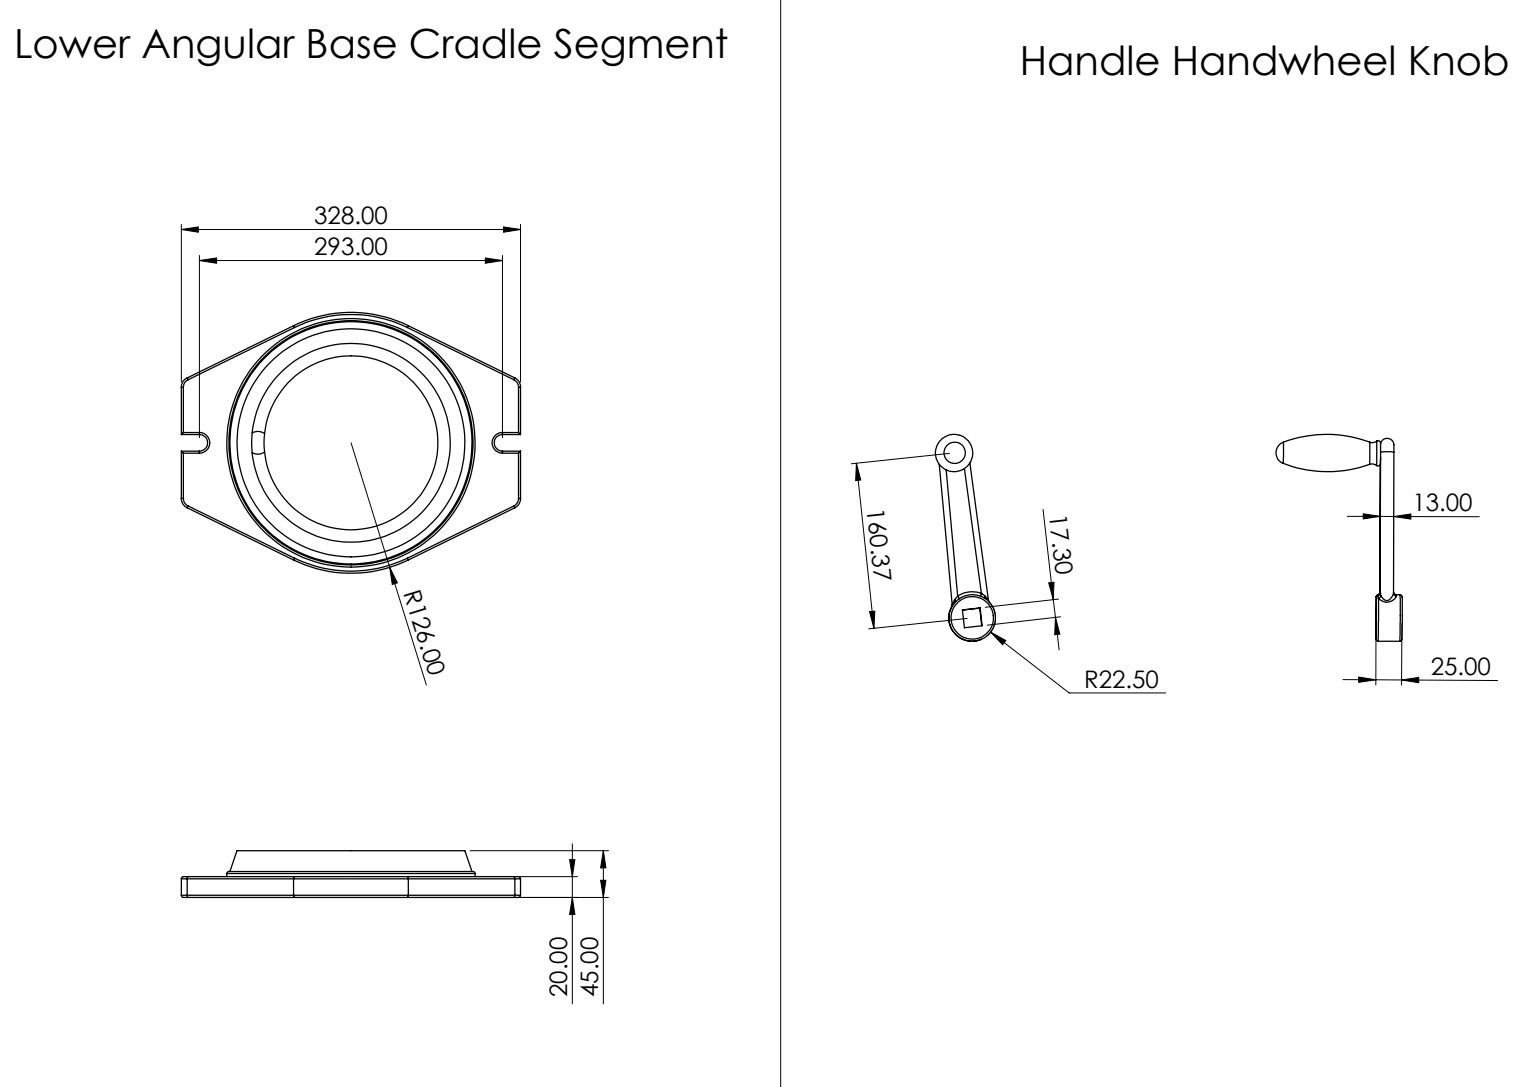
ISO-10303-21;
HEADER;
FILE_DESCRIPTION (('STEP AP214'),
    '1' );
FILE_NAME ('Handle Handwheel Knob.step',
    '2026-10-09T10:51:02',
    ( '' ),
    ( '' ),
    'SwSTEP 2.0',
    'SolidWorks 2026',
    '' );
FILE_SCHEMA (( 'AUTOMOTIVE_DESIGN' ));
ENDSEC;

DATA;
#6=CARTESIAN_POINT ( 'NONE',  ( -0.1662275214367944787, 327.2814318531398499, 311.3351636502816291 ) ) ;
#24=DIRECTION ( 'NONE',  ( 0.9935244165829104634, 0.1136188085379686713, 0.000000000000000000 ) ) ;
#26=CARTESIAN_POINT ( 'NONE',  ( -10.01057122740781402, 165.1012737418342056, 308.8014639846969089 ) ) ;
#27=EDGE_CURVE ( 'NONE', #4135, #17067, #5079, .T. ) ;
#41=CARTESIAN_POINT ( 'NONE',  ( 15.61516006123881795, 188.4668067408832144, 308.5202341143809690 ) ) ;
#52=CARTESIAN_POINT ( 'NONE',  ( 13.04681478898882219, 190.3009582326741622, 320.8498813576193243 ) ) ;
#55=CARTESIAN_POINT ( 'NONE',  ( 19.35063451732290929, 183.1639393726175058, 309.5798762404240847 ) ) ;
#63=CARTESIAN_POINT ( 'NONE',  ( -8.812762866403248907, 186.1645115285507188, 321.8620257335252859 ) ) ;
#87=CARTESIAN_POINT ( 'NONE',  ( -8.855655583235034101, 185.7709171679380802, 321.2465429934534313 ) ) ;
#92=DIRECTION ( 'NONE',  ( 0.9934404589540164476, 0.1135548637187057258, -0.01346653032743022095 ) ) ;
#97=CARTESIAN_POINT ( 'NONE',  ( -15.45047209318716419, 177.9595801977488634, 312.9923267615550344 ) ) ;
#100=B_SPLINE_CURVE_WITH_KNOTS ( 'NONE', 3,
 ( #8667, #13977, #4769, #10088, #15381, #20512, #13534 ),
 .UNSPECIFIED., .F., .F.,
 ( 4, 3, 4 ),
 ( -5.915969516749687466E-08, 0.000000000000000000, 2.978207829266907417E-05 ),
 .UNSPECIFIED. ) ;
#101=CARTESIAN_POINT ( 'NONE',  ( 17.83180013577688783, 184.4306634807684588, 307.6366520947308345 ) ) ;
#125=EDGE_CURVE ( 'NONE', #4735, #5612, #10337, .T. ) ;
#126=VERTEX_POINT ( 'NONE', #10448 ) ;
#128=CARTESIAN_POINT ( 'NONE',  ( 0.3194159855789066582, 327.3487718243365521, 314.2597695910868651 ) ) ;
#138=EDGE_CURVE ( 'NONE', #1183, #6442, #10411, .T. ) ;
#152=CARTESIAN_POINT ( 'NONE',  ( -28.12186643111994044, 324.0859723387359850, 311.7141148554663914 ) ) ;
#166=CARTESIAN_POINT ( 'NONE',  ( 14.63430001765469868, 189.2724070846429072, 308.1616490980433696 ) ) ;
#181=CARTESIAN_POINT ( 'NONE',  ( 15.18113699892158763, 188.8369998821271452, 308.3433818295962396 ) ) ;
#192=FACE_OUTER_BOUND ( 'NONE', #4432, .T. ) ;
#203=CARTESIAN_POINT ( 'NONE',  ( -8.718981069309306164, 185.8769606721263017, 321.2367416126799640 ) ) ;
#209=CARTESIAN_POINT ( 'NONE',  ( -16.46732747216173820, 164.3349221900030557, 301.8725943425079095 ) ) ;
#210=CARTESIAN_POINT ( 'NONE',  ( 15.90349308958513141, 168.0612899129591824, 307.9342904543644863 ) ) ;
#211=CARTESIAN_POINT ( 'NONE',  ( -13.46841022152523237, 180.7689078494431669, 321.2689861962914506 ) ) ;
#213=CARTESIAN_POINT ( 'NONE',  ( 20.69445389845595784, 181.8968845288082434, 314.6913679966366999 ) ) ;
#220=EDGE_CURVE ( 'NONE', #18203, #7136, #3541, .T. ) ;
#221=CARTESIAN_POINT ( 'NONE',  ( -17.10066205189340849, 316.2389990861104820, 322.8183011548654804 ) ) ;
#234=DIRECTION ( 'NONE',  ( -0.01292394549866745720, -0.005513023399720816918, -0.9999012842304692006 ) ) ;
#239=CARTESIAN_POINT ( 'NONE',  ( 21.90287145686899706, 168.7773271647431841, 315.3565719312696842 ) ) ;
#249=DIRECTION ( 'NONE',  ( 0.3101392564284310427, 0.9506461370142480494, -0.009250070373107139796 ) ) ;
#261=CARTESIAN_POINT ( 'NONE',  ( -28.28143568398816399, 324.0695986473149901, 312.1786345499324398 ) ) ;
#273=CARTESIAN_POINT ( 'NONE',  ( 19.91213793988244163, 183.5619383714575861, 314.9323046934921422 ) ) ;
#283=CARTESIAN_POINT ( 'NONE',  ( 19.70626577706693894, 182.8347090725441433, 310.2503944804881826 ) ) ;
#290=CARTESIAN_POINT ( 'NONE',  ( -9.470826101554981946, 187.1917151187963384, 321.2300099800097541 ) ) ;
#295=EDGE_LOOP ( 'NONE', ( #16677, #766, #19558, #3200 ) ) ;
#305=DIRECTION ( 'NONE',  ( 0.9506032891036977350, -0.3102281881984299550, -0.01057629388543066158 ) ) ;
#308=CARTESIAN_POINT ( 'NONE',  ( -22.02882225528089322, 319.7347194434814242, 320.5895957426023415 ) ) ;
#313=CARTESIAN_POINT ( 'NONE',  ( -10.06383400738342360, 187.4687485412983108, 321.1393786276795481 ) ) ;
#318=CARTESIAN_POINT ( 'NONE',  ( -13.33381189847107784, 183.5857969768588589, 309.7596506135559480 ) ) ;
#322=CARTESIAN_POINT ( 'NONE',  ( 18.31365161534814945, 168.3394720871181960, 308.5681747117120608 ) ) ;
#323=CARTESIAN_POINT ( 'NONE',  ( -14.60451153091767118, 179.2935387600311401, 317.4001766113444774 ) ) ;
#328=CARTESIAN_POINT ( 'NONE',  ( 11.85964614693714836, 187.7423844643599296, 304.8777488482054423 ) ) ;
#330=CARTESIAN_POINT ( 'NONE',  ( -9.841028579513169561, 187.8130746588807938, 321.1594247271215750 ) ) ;
#342=DIRECTION ( 'NONE',  ( 0.3101392564284315978, 0.9506461370142478273, -0.009250070373107145000 ) ) ;
#350=CARTESIAN_POINT ( 'NONE',  ( 0.2417370086904135351, 327.3338204178164688, 312.7560729848880214 ) ) ;
#360=CARTESIAN_POINT ( 'NONE',  ( -12.86548928906161571, 326.2291019854885121, 410.4442357137708086 ) ) ;
#372=CARTESIAN_POINT ( 'NONE',  ( -24.73308955485819283, 324.4589790655039110, 308.1131263010046837 ) ) ;
#382=ORIENTED_EDGE ( 'NONE', *, *, #15008, .F. ) ;
#385=CARTESIAN_POINT ( 'NONE',  ( 19.41596747074044060, 184.3392198334767329, 316.6735434663280557 ) ) ;
#399=CARTESIAN_POINT ( 'NONE',  ( 19.45541216839452048, 183.1297393420369417, 311.7642400163919660 ) ) ;
#408=CARTESIAN_POINT ( 'NONE',  ( -8.586490856789254167, 185.8024398487989686, 322.3033838124611634 ) ) ;
#431=CARTESIAN_POINT ( 'NONE',  ( -9.125680706444326162, 185.5535976647744860, 321.2577656795050984 ) ) ;
#435=CARTESIAN_POINT ( 'NONE',  ( -13.42037733046067238, 183.2664398413913887, 319.4772174752336582 ) ) ;
#439=CARTESIAN_POINT ( 'NONE',  ( -15.18250214363469119, 179.4876624324358261, 314.9100870799183554 ) ) ;
#504=CARTESIAN_POINT ( 'NONE',  ( 19.56830941617827335, 184.1114337889866874, 316.3329861247396479 ) ) ;
#518=CARTESIAN_POINT ( 'NONE',  ( 19.38763582148057907, 184.2660337520671590, 312.0117097956302814 ) ) ;
#538=CARTESIAN_POINT ( 'NONE',  ( 4.169604791867612015, 166.7785703876306513, 322.5944574396354483 ) ) ;
#553=CARTESIAN_POINT ( 'NONE',  ( -15.17867682233058524, 179.5161877312053207, 314.3080855853813205 ) ) ;
#556=DIRECTION ( 'NONE',  ( -0.9935244165829104634, -0.1136188085379686713, 0.000000000000000000 ) ) ;
#557=CARTESIAN_POINT ( 'NONE',  ( -15.13164630670634736, 179.6607342462910708, 313.7313605305386091 ) ) ;
#565=DIRECTION ( 'NONE',  ( 0.9934404589540163366, 0.1135548637187057675, -0.01346653032742958604 ) ) ;
#596=DIRECTION ( 'NONE',  ( -0.01292394549866742424, -0.005513023399720750999, -0.9999012842304693116 ) ) ;
#628=CARTESIAN_POINT ( 'NONE',  ( 18.96776859854577069, 184.9744126260587791, 317.4480445392455294 ) ) ;
#637=EDGE_CURVE ( 'NONE', #13714, #126, #15945, .T. ) ;
#642=CARTESIAN_POINT ( 'NONE',  ( -12.58664483627419095, 184.6272112293399630, 320.1917372557430213 ) ) ;
#658=CARTESIAN_POINT ( 'NONE',  ( -8.575531608407624518, 185.9784460181284089, 321.2405749393824976 ) ) ;
#662=CARTESIAN_POINT ( 'NONE',  ( -14.79896642201964418, 180.4272692235275315, 317.1363243735250421 ) ) ;
#664=CARTESIAN_POINT ( 'NONE',  ( -9.822685604078287724, 184.4798924047493642, 305.4113335104130442 ) ) ;
#667=ORIENTED_EDGE ( 'NONE', *, *, #3510, .T. ) ;
#674=CARTESIAN_POINT ( 'NONE',  ( 12.48881921303416398, 189.6164759944761897, 307.6758311242440982 ) ) ;
#730=CARTESIAN_POINT ( 'NONE',  ( 13.58462956591013615, 190.0212252665789094, 307.9296231100185537 ) ) ;
#734=MECHANICAL_DESIGN_GEOMETRIC_PRESENTATION_REPRESENTATION('',(#10620),#15073);
#746=CARTESIAN_POINT ( 'NONE',  ( 19.93997345945722799, 182.7315227521808936, 315.6546791933524787 ) ) ;
#766=ORIENTED_EDGE ( 'NONE', *, *, #125, .T. ) ;
#782=CARTESIAN_POINT ( 'NONE',  ( -9.048035673407987645, 185.0480505508585907, 307.9947944869788898 ) ) ;
#799=CARTESIAN_POINT ( 'NONE',  ( -14.20436985759224235, 179.8017517255571818, 320.1469751989672545 ) ) ;
#809=AXIS2_PLACEMENT_3D ( 'NONE', #3079, #12155, #12280 ) ;
#810=CARTESIAN_POINT ( 'NONE',  ( -8.564669286038160578, 185.5585649246744140, 306.1008109505842754 ) ) ;
#826=FACE_BOUND ( 'NONE', #21834, .T. ) ;
#838=CARTESIAN_POINT ( 'NONE',  ( -7.810477471022748475, 165.3506309087785553, 308.2453597648303685 ) ) ;
#846=CARTESIAN_POINT ( 'NONE',  ( 11.80591785795528104, 176.3657631373681056, 324.4430942173937638 ) ) ;
#854=B_SPLINE_CURVE_WITH_KNOTS ( 'NONE', 3,
 ( #18218, #21952, #12942, #4063, #16834, #5778, #2583 ),
 .UNSPECIFIED., .F., .F.,
 ( 4, 3, 4 ),
 ( 0.000000000000000000, 3.076089232684222182E-05, 3.082002332305258858E-05 ),
 .UNSPECIFIED. ) ;
#869=CARTESIAN_POINT ( 'NONE',  ( 18.86594229807002421, 185.1130985469481800, 317.5966198224662094 ) ) ;
#871=CARTESIAN_POINT ( 'NONE',  ( -3.415012492225389273, 157.2134297314921128, 324.7454257987990331 ) ) ;
#902=CARTESIAN_POINT ( 'NONE',  ( -12.78366430685853672, 181.7268150396907345, 309.3689789245013344 ) ) ;
#908=CARTESIAN_POINT ( 'NONE',  ( 11.85847056065619221, 187.7666840159210437, 305.2629551530478125 ) ) ;
#917=ORIENTED_EDGE ( 'NONE', *, *, #10755, .T. ) ;
#921=DIRECTION ( 'NONE',  ( 0.01292394549866727679, 0.005513023399720742325, 0.9999012842304692006 ) ) ;
#933=ORIENTED_EDGE ( 'NONE', *, *, #14009, .T. ) ;
#939=DIRECTION ( 'NONE',  ( -0.9934404589540161146, -0.1135548637187070442, 0.01346653032743022269 ) ) ;
#973=CARTESIAN_POINT ( 'NONE',  ( 24.23788345395560384, 168.9796455556705723, 299.3206640306223676 ) ) ;
#974=CARTESIAN_POINT ( 'NONE',  ( 17.82481991809018140, 186.4251367409188163, 318.7777147611763553 ) ) ;
#975=ADVANCED_FACE ( 'NONE', ( #17419 ), #6180, .T. ) ;
#981=DIRECTION ( 'NONE',  ( 0.1136178953597579561, -0.9935164314186356593, 0.004009283626633663132 ) ) ;
#1001=ADVANCED_FACE ( 'NONE', ( #19114 ), #14443, .F. ) ;
#1007=CARTESIAN_POINT ( 'NONE',  ( -11.47056600305460350, 183.0990483233374846, 308.4747080909204442 ) ) ;
#1010=CARTESIAN_POINT ( 'NONE',  ( 12.16442896649338223, 187.7168230983759543, 322.9757373289252200 ) ) ;
#1020=CARTESIAN_POINT ( 'NONE',  ( 12.21805463999710817, 187.9383611531376914, 322.3984907411651193 ) ) ;
#1067=CARTESIAN_POINT ( 'NONE',  ( -5.563703806604336499, 326.7005119474492290, 320.3383740725300299 ) ) ;
#1077=CARTESIAN_POINT ( 'NONE',  ( -17.21821209452539847, 315.6014859805258652, 330.9526324688387717 ) ) ;
#1083=CARTESIAN_POINT ( 'NONE',  ( 17.83341159513771856, 184.6399546625437722, 321.1738318148023836 ) ) ;
#1108=DIRECTION ( 'NONE',  ( -0.01292394549866727679, -0.005513023399720743192, -0.9999012842304693116 ) ) ;
#1109=CARTESIAN_POINT ( 'NONE',  ( 12.82628922073134170, 190.6145596806321407, 307.8497150165550238 ) ) ;
#1125=CARTESIAN_POINT ( 'NONE',  ( -13.62391555017718048, 183.0616513303022543, 310.0861352889502314 ) ) ;
#1140=DIRECTION ( 'NONE',  ( 0.3101392564284315978, 0.9506461370142478273, -0.009250070373107145000 ) ) ;
#1164=DIRECTION ( 'NONE',  ( -0.9934404589540163366, -0.1135548637187060866, 0.01346653032743036840 ) ) ;
#1183=VERTEX_POINT ( 'NONE', #1864 ) ;
#1205=ORIENTED_EDGE ( 'NONE', *, *, #10755, .F. ) ;
#1206=CARTESIAN_POINT ( 'NONE',  ( -16.17007672569239318, 164.4617217281966361, 324.8703238798086659 ) ) ;
#1208=CARTESIAN_POINT ( 'NONE',  ( 15.97866707245144902, 185.9292776491716381, 320.3317121505914997 ) ) ;
#1216=DIRECTION ( 'NONE',  ( -0.9934404589540162256, -0.1135548637187057258, 0.01346653032743021748 ) ) ;
#1224=ORIENTED_EDGE ( 'NONE', *, *, #8533, .T. ) ;
#1247=CARTESIAN_POINT ( 'NONE',  ( -9.772617557124883447, 188.0380679982199581, 308.1349344327151130 ) ) ;
#1248=EDGE_LOOP ( 'NONE', ( #10587, #8874 ) ) ;
#1255=CARTESIAN_POINT ( 'NONE',  ( 14.00406913739424830, 186.9630538133311006, 322.8218460857456193 ) ) ;
#1258=CARTESIAN_POINT ( 'NONE',  ( -0.3844496095692996329, 327.2789202713466352, 316.8969144942429921 ) ) ;
#1264=VERTEX_POINT ( 'NONE', #11052 ) ;
#1265=CARTESIAN_POINT ( 'NONE',  ( 12.29214828332425924, 188.1889653831995020, 322.0203645085242670 ) ) ;
#1281=ORIENTED_EDGE ( 'NONE', *, *, #11747, .T. ) ;
#1352=CARTESIAN_POINT ( 'NONE',  ( -10.17049351323417561, 187.7283718258219949, 308.1773159039984762 ) ) ;
#1357=CARTESIAN_POINT ( 'NONE',  ( 16.40873467035000033, 185.6567299720572635, 322.3321779654820602 ) ) ;
#1364=CARTESIAN_POINT ( 'NONE',  ( 13.70891000273312343, 189.9149113544312399, 320.7681615485908537 ) ) ;
#1368=FACE_OUTER_BOUND ( 'NONE', #21089, .T. ) ;
#1370=EDGE_CURVE ( 'NONE', #19478, #5262, #3205, .T. ) ;
#1374=CARTESIAN_POINT ( 'NONE',  ( -16.19592461668972661, 164.4506956813972067, 322.8705213113477726 ) ) ;
#1376=CARTESIAN_POINT ( 'NONE',  ( -12.01575389182678499, 182.4076787623492066, 322.7174846376903474 ) ) ;
#1378=CARTESIAN_POINT ( 'NONE',  ( -25.68841619517593955, 324.3516952872404318, 308.6004965912300690 ) ) ;
#1395=DIRECTION ( 'NONE',  ( 1.000000000000000000, 0.000000000000000000, 0.000000000000000000 ) ) ;
#1399=AXIS2_PLACEMENT_3D ( 'NONE', #7003, #12191, #342 ) ;
#1450=CARTESIAN_POINT ( 'NONE',  ( 13.01890817498768449, 190.3110758050131892, 320.8522954438618058 ) ) ;
#1472=CARTESIAN_POINT ( 'NONE',  ( 13.55544375494392817, 190.0065045115472913, 320.7925508485532760 ) ) ;
#1480=FACE_OUTER_BOUND ( 'NONE', #8854, .T. ) ;
#1503=ORIENTED_EDGE ( 'NONE', *, *, #12891, .T. ) ;
#1548=TOROIDAL_SURFACE ( 'NONE', #1905, 20.50000000000000355, 2.000000000000000000 ) ;
#1560=CARTESIAN_POINT ( 'NONE',  ( 11.78290328754079219, 187.7711080693391921, 304.8720351003711357 ) ) ;
#1578=SPHERICAL_SURFACE ( 'NONE', #14052, 11.00000000000000533 ) ;
#1594=CARTESIAN_POINT ( 'NONE',  ( 14.92693155316947262, 186.3292256045772604, 305.6379776027275170 ) ) ;
#1632=DIRECTION ( 'NONE',  ( -0.01292394549866727679, -0.005513023399720742325, -0.9999012842304692006 ) ) ;
#1634=ADVANCED_FACE ( 'NONE', ( #19289 ), #5393, .F. ) ;
#1648=DIRECTION ( 'NONE',  ( 0.1136178953597579561, -0.9935164314186356593, 0.004009283626633663132 ) ) ;
#1651=VECTOR ( 'NONE', #15859, 999.9999999999998863 ) ;
#1661=ORIENTED_EDGE ( 'NONE', *, *, #3227, .T. ) ;
#1675=( NAMED_UNIT ( * ) PLANE_ANGLE_UNIT ( ) SI_UNIT ( $, .RADIAN. ) );
#1678=CARTESIAN_POINT ( 'NONE',  ( 11.82873084905181749, 187.7848449878356405, 307.7666980689497791 ) ) ;
#1691=DIRECTION ( 'NONE',  ( -0.01292394549866745720, -0.005513023399720816918, -0.9999012842304692006 ) ) ;
#1708=CARTESIAN_POINT ( 'NONE',  ( 20.16650508637343719, 182.5115947525307263, 317.5179922051294739 ) ) ;
#1734=CARTESIAN_POINT ( 'NONE',  ( 0.3064506171779977084, 327.3432411309900090, 313.2566634950479170 ) ) ;
#1740=ORIENTED_EDGE ( 'NONE', *, *, #7164, .T. ) ;
#1754=CARTESIAN_POINT ( 'NONE',  ( -8.905365697803494740, 165.2773500475165065, 321.1137824091954940 ) ) ;
#1775=CARTESIAN_POINT ( 'NONE',  ( -14.02864438394168722, 325.7329298795136197, 320.4531201330285626 ) ) ;
#1780=CARTESIAN_POINT ( 'NONE',  ( 14.12971913360413367, 189.6478225779368358, 308.0282301501843563 ) ) ;
#1798=ORIENTED_EDGE ( 'NONE', *, *, #5168, .F. ) ;
#1802=CIRCLE ( 'NONE', #11336, 22.50000000000000000 ) ;
#1805=CARTESIAN_POINT ( 'NONE',  ( -12.19462927199251112, 185.2216277673267939, 320.4682053348163890 ) ) ;
#1811=DIRECTION ( 'NONE',  ( -0.7193492748294019190, 0.6946270388778962301, 0.005467875468530753770 ) ) ;
#1813=CARTESIAN_POINT ( 'NONE',  ( 15.81758052762976341, 168.0514417711093529, 307.9285322505227782 ) ) ;
#1814=CARTESIAN_POINT ( 'NONE',  ( -15.16114907798143285, 179.5344160342980615, 315.3037902903944314 ) ) ;
#1822=ADVANCED_FACE ( 'NONE', ( #192 ), #4319, .F. ) ;
#1840=CARTESIAN_POINT ( 'NONE',  ( 15.98577074487546312, 168.1231874004433280, 320.9410920942888197 ) ) ;
#1845=ORIENTED_EDGE ( 'NONE', *, *, #21487, .T. ) ;
#1864=CARTESIAN_POINT ( 'NONE',  ( -10.32533161609876871, 336.9590297039326288, 324.0204083566396207 ) ) ;
#1865=CARTESIAN_POINT ( 'NONE',  ( -7.642197790895533416, 165.4224147006813155, 321.2648411829814563 ) ) ;
#1882=CARTESIAN_POINT ( 'NONE',  ( 15.29545575833136084, 188.7412618571948144, 308.3876529512198204 ) ) ;
#1893=CARTESIAN_POINT ( 'NONE',  ( 13.03751462902003055, 190.3043364584464143, 320.8506857707324684 ) ) ;
#1896=CARTESIAN_POINT ( 'NONE',  ( 16.47746874666049166, 185.3946093038764218, 306.5053848239848548 ) ) ;
#1902=CARTESIAN_POINT ( 'NONE',  ( -9.012827358357725416, 186.4798162552521603, 321.5937060577796842 ) ) ;
#1905=AXIS2_PLACEMENT_3D ( 'NONE', #16224, #921, #17933 ) ;
#1911=AXIS2_PLACEMENT_3D ( 'NONE', #7697, #5853, #21910 ) ;
#1921=CARTESIAN_POINT ( 'NONE',  ( 12.33097383755215937, 187.6544282282688414, 322.9682109676994628 ) ) ;
#1927=CARTESIAN_POINT ( 'NONE',  ( -9.866459160504181369, 187.6519449355448046, 321.1574017861566972 ) ) ;
#1931=CARTESIAN_POINT ( 'NONE',  ( -15.16562817910661387, 179.5584899311543552, 314.0881026776677345 ) ) ;
#1934=CARTESIAN_POINT ( 'NONE',  ( -5.731715098087012628, 326.6288426432528240, 307.3396573775339107 ) ) ;
#1935=CARTESIAN_POINT ( 'NONE',  ( -13.94857819362903939, 180.2051281715647804, 318.6524844431677934 ) ) ;
#1937=CARTESIAN_POINT ( 'NONE',  ( 19.54762674317498039, 182.9836852283762880, 309.9251239444264456 ) ) ;
#1943=ORIENTED_EDGE ( 'NONE', *, *, #18930, .F. ) ;
#1965=CARTESIAN_POINT ( 'NONE',  ( 18.46443518240318937, 168.4037924862991815, 320.2340148651496179 ) ) ;
#1967=VERTEX_POINT ( 'NONE', #6596 ) ;
#1974=ORIENTED_EDGE ( 'NONE', *, *, #19587, .T. ) ;
#1988=CARTESIAN_POINT ( 'NONE',  ( -12.65694952506544801, 164.8377797042643635, 318.5015202093982225 ) ) ;
#1996=ORIENTED_EDGE ( 'NONE', *, *, #8299, .F. ) ;
#2008=AXIS2_PLACEMENT_3D ( 'NONE', #10847, #16145, #21169 ) ;
#2013=CARTESIAN_POINT ( 'NONE',  ( 18.63884989169994100, 183.8434042675073954, 310.4714192387435787 ) ) ;
#2031=CARTESIAN_POINT ( 'NONE',  ( 12.21332820092900739, 188.3547093575519682, 320.9587726345017131 ) ) ;
#2041=CARTESIAN_POINT ( 'NONE',  ( -14.34866974388063099, 181.6106202444769906, 311.1517963829039104 ) ) ;
#2044=CARTESIAN_POINT ( 'NONE',  ( -15.06566084134985850, 178.6016716131798887, 315.4181938385037256 ) ) ;
#2095=CARTESIAN_POINT ( 'NONE',  ( -26.01799913968005384, 324.3151495388358967, 308.8842677255468061 ) ) ;
#2115=CARTESIAN_POINT ( 'NONE',  ( 13.58411996604009886, 190.0215289310135347, 307.9295376775164073 ) ) ;
#2122=ORIENTED_EDGE ( 'NONE', *, *, #8358, .T. ) ;
#2133=CARTESIAN_POINT ( 'NONE',  ( 12.23821171205838709, 188.3449730651813638, 320.9566317594674274 ) ) ;
#2136=LINE ( 'NONE', #12384, #22139 ) ;
#2139=CARTESIAN_POINT ( 'NONE',  ( -9.651817171046198851, 185.0982321658034948, 321.2476234092152367 ) ) ;
#2144=CARTESIAN_POINT ( 'NONE',  ( -15.18631308743390740, 179.4818830208618010, 314.7524899164025101 ) ) ;
#2145=ORIENTED_EDGE ( 'NONE', *, *, #4888, .F. ) ;
#2148=CARTESIAN_POINT ( 'NONE',  ( -14.75085724879592419, 179.0757283420780936, 316.9950527168435883 ) ) ;
#2152=DIRECTION ( 'NONE',  ( -0.9934404589540165587, -0.1135548637187044907, 0.01346653032743213955 ) ) ;
#2186=TOROIDAL_SURFACE ( 'NONE', #5103, 17.29295143883736330, 7.000000000000003553 ) ;
#2188=AXIS2_PLACEMENT_3D ( 'NONE', #17082, #6393, #3045 ) ;
#2190=EDGE_CURVE ( 'NONE', #13179, #3953, #100, .T. ) ;
#2194=DIRECTION ( 'NONE',  ( -0.01292394549866745720, -0.005513023399720816918, -0.9999012842304692006 ) ) ;
#2197=CARTESIAN_POINT ( 'NONE',  ( -28.53175067654398234, 324.0509493238391201, 314.6508600760126910 ) ) ;
#2213=CARTESIAN_POINT ( 'NONE',  ( 17.50001040944635378, 186.7960900973744742, 319.0550816609377875 ) ) ;
#2219=DIRECTION ( 'NONE',  ( -0.9506868100732489557, 0.3101525256269085928, 0.000000000000000000 ) ) ;
#2225=CARTESIAN_POINT ( 'NONE',  ( 12.89457967643548031, 187.3266554051253081, 305.0022774674998800 ) ) ;
#2227=AXIS2_PLACEMENT_3D ( 'NONE', #13603, #8077, #20588 ) ;
#2232=DIRECTION ( 'NONE',  ( -0.01292394549866754394, -0.005513023399720772683, -0.9999012842304692006 ) ) ;
#2263=AXIS2_PLACEMENT_3D ( 'NONE', #17479, #234, #13903 ) ;
#2271=CARTESIAN_POINT ( 'NONE',  ( -15.06976562345401227, 178.6172216735134555, 313.9837765850090250 ) ) ;
#2287=DIRECTION ( 'NONE',  ( -0.01292394549866745720, -0.005513023399720816918, -0.9999012842304692006 ) ) ;
#2348=CARTESIAN_POINT ( 'NONE',  ( 20.58420809267111196, 182.0421985228920505, 315.9315213838523846 ) ) ;
#2388=CARTESIAN_POINT ( 'NONE',  ( -10.03308090247307405, 188.0016273849522861, 308.1595840160059083 ) ) ;
#2390=CARTESIAN_POINT ( 'NONE',  ( -14.90497309951318883, 180.1700006406394436, 316.7981750502078171 ) ) ;
#2394=CARTESIAN_POINT ( 'NONE',  ( -13.80640766535087849, 180.4787919979394530, 308.4662719087184541 ) ) ;
#2418=CARTESIAN_POINT ( 'NONE',  ( -9.995692194476635706, 187.8898849410517471, 308.1575541326492953 ) ) ;
#2458=CARTESIAN_POINT ( 'NONE',  ( 20.03694923833142028, 182.5980394464318408, 313.7561223232668794 ) ) ;
#2496=CARTESIAN_POINT ( 'NONE',  ( -12.36665144395150762, 182.1817021327200621, 309.0434142697981770 ) ) ;
#2504=B_SPLINE_CURVE_WITH_KNOTS ( 'NONE', 3,
 ( #1357, #18679, #17097, #1255, #18578, #22221, #20631, #1010 ),
 .UNSPECIFIED., .F., .F.,
 ( 4, 2, 2, 4 ),
 ( 0.000000000000000000, 0.002382335671685098782, 0.003573503507527667905, 0.004764671343370237462 ),
 .UNSPECIFIED. ) ;
#2511=CARTESIAN_POINT ( 'NONE',  ( -12.68046251919286149, 181.8339994666508233, 307.1133876553329856 ) ) ;
#2522=CARTESIAN_POINT ( 'NONE',  ( -8.523216527044569446, 185.4125284852929099, 305.1540476800932424 ) ) ;
#2529=B_SPLINE_CURVE_WITH_KNOTS ( 'NONE', 3,
 ( #15362, #6601, #13629, #1450 ),
 .UNSPECIFIED., .F., .F.,
 ( 4, 4 ),
 ( 2.775557561562891351E-17, 0.0001171670690882713705 ),
 .UNSPECIFIED. ) ;
#2556=B_SPLINE_CURVE_WITH_KNOTS ( 'NONE', 3,
 ( #9400, #7573, #5615, #11253, #21665, #14605, #21557, #5832, #4110, #5957, #1265, #1020, #13103, #15390 ),
 .UNSPECIFIED., .F., .F.,
 ( 4, 2, 2, 2, 2, 2, 4 ),
 ( 0.000000000000000000, 0.0009165371227101086048, 0.001374805684065199445, 0.001833074245420290502, 0.002291342806775381342, 0.002749611368130472182, 0.003666148490840745369 ),
 .UNSPECIFIED. ) ;
#2575=CARTESIAN_POINT ( 'NONE',  ( 19.53622439867276128, 183.1519941725404408, 318.8984196516840370 ) ) ;
#2583=CARTESIAN_POINT ( 'NONE',  ( -10.02117361870881851, 187.8727420016839176, 308.1601407300097435 ) ) ;
#2589=VECTOR ( 'NONE', #13773, 999.9999999999998863 ) ;
#2598=CARTESIAN_POINT ( 'NONE',  ( -3.414999568279890152, 157.2134352445154946, 324.7464257000832504 ) ) ;
#2606=CIRCLE ( 'NONE', #16563, 10.29357798165139393 ) ;
#2613=CARTESIAN_POINT ( 'NONE',  ( -8.886709464532664526, 185.1602439857121283, 307.9998212653392784 ) ) ;
#2631=CARTESIAN_POINT ( 'NONE',  ( -10.22841750353083334, 184.1639157294440565, 305.5386342265414896 ) ) ;
#2643=VERTEX_POINT ( 'NONE', #11151 ) ;
#2644=CIRCLE ( 'NONE', #2263, 10.29295143883735619 ) ;
#2657=AXIS2_PLACEMENT_3D ( 'NONE', #7588, #19862, #10700 ) ;
#2677=CARTESIAN_POINT ( 'NONE',  ( 12.84378735233264379, 190.4863133572641232, 307.8501959441126701 ) ) ;
#2697=CARTESIAN_POINT ( 'NONE',  ( 20.06878510934510729, 182.5747025716839289, 314.2333932023548186 ) ) ;
#2700=VECTOR ( 'NONE', #16303, 999.9999999999998863 ) ;
#2714=DIRECTION ( 'NONE',  ( 0.01292394549866727679, 0.005513023399720742325, 0.9999012842304692006 ) ) ;
#2730=CARTESIAN_POINT ( 'NONE',  ( 12.81503532323078964, 190.4972571607467842, 307.8483445055002221 ) ) ;
#2731=CARTESIAN_POINT ( 'NONE',  ( -13.29639799380280074, 181.1157429896730946, 307.7937712325852999 ) ) ;
#2744=CARTESIAN_POINT ( 'NONE',  ( 3.212670811948540095, 175.3835190792246976, 324.5605796060102648 ) ) ;
#2749=PLANE ( 'NONE',  #11819 ) ;
#2766=DIRECTION ( 'NONE',  ( 0.01292394549866727853, 0.005513023399720741458, 0.9999012842304692006 ) ) ;
#2802=CARTESIAN_POINT ( 'NONE',  ( 20.39811478720299220, 182.2549943958479446, 316.7388195023896742 ) ) ;
#2834=CARTESIAN_POINT ( 'NONE',  ( -12.67437722926222143, 184.6792686180227179, 309.1546888890629816 ) ) ;
#2845=DIRECTION ( 'NONE',  ( 0.1136178953597579561, -0.9935164314186356593, 0.004009283626633661397 ) ) ;
#2855=AXIS2_PLACEMENT_3D ( 'NONE', #20215, #4481, #11512 ) ;
#2880=CARTESIAN_POINT ( 'NONE',  ( 18.04061865414768207, 188.1738179166474367, 322.2972073689282979 ) ) ;
#2907=CARTESIAN_POINT ( 'NONE',  ( 16.39634482804412130, 187.9401017119209882, 319.7988598509798521 ) ) ;
#2929=DIRECTION ( 'NONE',  ( 0.09199399308265900077, -0.9957502728239346901, 0.004301093787334644286 ) ) ;
#2952=CARTESIAN_POINT ( 'NONE',  ( 15.62064282387096092, 186.1419012809308526, 320.4776025279708733 ) ) ;
#2969=CARTESIAN_POINT ( 'NONE',  ( -28.54870338537778096, 324.0437177334164858, 313.3392609721734061 ) ) ;
#2983=CARTESIAN_POINT ( 'NONE',  ( -8.562029719258356764, 342.2165115496170529, 328.2923693891043513 ) ) ;
#3002=CIRCLE ( 'NONE', #2657, 7.000000000000022204 ) ;
#3020=CARTESIAN_POINT ( 'NONE',  ( 16.40873467034967703, 185.6567299720570645, 322.3321779654822876 ) ) ;
#3027=CARTESIAN_POINT ( 'NONE',  ( -12.58664483627419095, 184.6272112293399630, 320.1917372557430213 ) ) ;
#3045=DIRECTION ( 'NONE',  ( 0.3101392564284313202, 0.9506461370142480494, -0.009250070373107143265 ) ) ;
#3064=ADVANCED_FACE ( 'NONE', ( #19265 ), #4587, .T. ) ;
#3071=DIRECTION ( 'NONE',  ( -0.01292394549866745720, -0.005513023399720816918, -0.9999012842304692006 ) ) ;
#3072=CIRCLE ( 'NONE', #4542, 1.999999999999998224 ) ;
#3079=CARTESIAN_POINT ( 'NONE',  ( 4.169604791867612015, 166.7785703876306513, 322.5944574396354483 ) ) ;
#3087=CIRCLE ( 'NONE', #13400, 22.49999999999999645 ) ;
#3090=CIRCLE ( 'NONE', #6760, 22.40787840283382693 ) ;
#3095=DIRECTION ( 'NONE',  ( -0.01292394549866754394, -0.005513023399720772683, -0.9999012842304692006 ) ) ;
#3102=CARTESIAN_POINT ( 'NONE',  ( 0.000000000000000000, 0.000000000000000000, 0.000000000000000000 ) ) ;
#3104=CIRCLE ( 'NONE', #14882, 10.29295143883735619 ) ;
#3121=CARTESIAN_POINT ( 'NONE',  ( -11.47153213676876859, 182.9699874009099858, 322.8803889165183136 ) ) ;
#3138=AXIS2_PLACEMENT_3D ( 'NONE', #15898, #10250, #12331 ) ;
#3139=CARTESIAN_POINT ( 'NONE',  ( -10.34796365319335543, 187.1999046744221857, 321.1016630495802815 ) ) ;
#3159=CARTESIAN_POINT ( 'NONE',  ( -10.05250806467569546, 187.8426943151429498, 308.1634901438939664 ) ) ;
#3170=VERTEX_POINT ( 'NONE', #3999 ) ;
#3176=VERTEX_POINT ( 'NONE', #2418 ) ;
#3200=ORIENTED_EDGE ( 'NONE', *, *, #19412, .F. ) ;
#3205=CIRCLE ( 'NONE', #2855, 22.50000000000000000 ) ;
#3227=EDGE_CURVE ( 'NONE', #17055, #3176, #6371, .T. ) ;
#3234=CARTESIAN_POINT ( 'NONE',  ( -5.380602081949200866, 174.4012639950344976, 324.6760651920582745 ) ) ;
#3260=ORIENTED_EDGE ( 'NONE', *, *, #20639, .F. ) ;
#3280=CARTESIAN_POINT ( 'NONE',  ( 13.24628194959730010, 190.1869353459286174, 320.8311507295203455 ) ) ;
#3292=DIRECTION ( 'NONE',  ( -0.9935244165829104634, -0.1136188085379686713, 0.000000000000000000 ) ) ;
#3296=CARTESIAN_POINT ( 'NONE',  ( 19.05734566456921542, 183.6057529188165915, 319.6991620761616559 ) ) ;
#3336=CARTESIAN_POINT ( 'NONE',  ( -5.027868580402196308, 326.7615858019005373, 320.2878431667282371 ) ) ;
#3343=EDGE_CURVE ( 'NONE', #4020, #17682, #17892, .T. ) ;
#3345=FACE_OUTER_BOUND ( 'NONE', #13519, .T. ) ;
#3385=CARTESIAN_POINT ( 'NONE',  ( 12.83141560359293898, 190.4910289390495279, 307.8493993209711448 ) ) ;
#3396=CARTESIAN_POINT ( 'NONE',  ( -8.819172402740010241, 185.2124387659711999, 305.1895671936096619 ) ) ;
#3400=EDGE_CURVE ( 'NONE', #2643, #17518, #20865, .T. ) ;
#3402=CARTESIAN_POINT ( 'NONE',  ( -14.02864438394168722, 325.7329298795136197, 320.4531201330285626 ) ) ;
#3424=VECTOR ( 'NONE', #11440, 1000.000000000000000 ) ;
#3425=CARTESIAN_POINT ( 'NONE',  ( 20.69883497493187718, 181.8866873879648267, 314.4189726352637990 ) ) ;
#3426=CARTESIAN_POINT ( 'NONE',  ( 13.77152037162459308, 159.1779343868491026, 324.5134547254186828 ) ) ;
#3454=CARTESIAN_POINT ( 'NONE',  ( 19.42790726798621748, 168.5114881856995623, 319.6178889223443775 ) ) ;
#3462=CARTESIAN_POINT ( 'NONE',  ( 5.178260401672350355, 158.1956848156823128, 324.6299402127509666 ) ) ;
#3468=DIRECTION ( 'NONE',  ( -0.01292394549866745720, -0.005513023399720816918, -0.9999012842304692006 ) ) ;
#3474=ORIENTED_EDGE ( 'NONE', *, *, #19142, .F. ) ;
#3477=CARTESIAN_POINT ( 'NONE',  ( -12.99577148999190612, 164.7709424335249366, 311.5407534607413709 ) ) ;
#3490=CARTESIAN_POINT ( 'NONE',  ( 18.76377268095312090, 185.1009473783541068, 310.9749437967080326 ) ) ;
#3500=CARTESIAN_POINT ( 'NONE',  ( 12.88272372176025016, 190.4631953211766131, 307.8527186633484121 ) ) ;
#3510=EDGE_CURVE ( 'NONE', #4020, #8155, #13945, .T. ) ;
#3516=DIRECTION ( 'NONE',  ( -0.3101392564284290998, -0.9506461370142487155, 0.009250070373107117244 ) ) ;
#3525=CARTESIAN_POINT ( 'NONE',  ( -10.61849163981879762, 184.1265005819461464, 321.1111245915606105 ) ) ;
#3541=LINE ( 'NONE', #10555, #7251 ) ;
#3560=CARTESIAN_POINT ( 'NONE',  ( 18.14299768316436001, 168.3676586590315765, 320.3890303468865000 ) ) ;
#3571=PLANE ( 'NONE',  #3138 ) ;
#3580=CARTESIAN_POINT ( 'NONE',  ( -24.57841208749768924, 324.5249605026011182, 320.0802301758413364 ) ) ;
#3593=CARTESIAN_POINT ( 'NONE',  ( 19.06930845108338701, 184.8361062471226717, 317.3053272177560871 ) ) ;
#3604=CARTESIAN_POINT ( 'NONE',  ( 14.21959016068815274, 186.7523085471082709, 307.8325657923471681 ) ) ;
#3608=EDGE_CURVE ( 'NONE', #19550, #8739, #20586, .T. ) ;
#3631=CARTESIAN_POINT ( 'NONE',  ( -12.01575389182707632, 182.4076787623489793, 322.7174846376827873 ) ) ;
#3633=CARTESIAN_POINT ( 'NONE',  ( -13.36217923100928928, 326.0172268059896510, 372.0162718331554288 ) ) ;
#3637=CARTESIAN_POINT ( 'NONE',  ( -12.26418779587024588, 185.2816307007135492, 308.8815972836887340 ) ) ;
#3640=CARTESIAN_POINT ( 'NONE',  ( -12.58827034560151681, 181.8529111828999589, 320.1441755304902586 ) ) ;
#3641=CARTESIAN_POINT ( 'NONE',  ( 12.36154785051915894, 187.5489770926929793, 304.9204778021706375 ) ) ;
#3658=ORIENTED_EDGE ( 'NONE', *, *, #14168, .T. ) ;
#3662=CARTESIAN_POINT ( 'NONE',  ( -5.731715098087014404, 326.6288426432528240, 307.3396573775339107 ) ) ;
#3664=AXIS2_PLACEMENT_3D ( 'NONE', #6016, #16384, #16275 ) ;
#3669=CARTESIAN_POINT ( 'NONE',  ( -2.207300919685918128, 327.0790409159932892, 319.0232558455138587 ) ) ;
#3690=CARTESIAN_POINT ( 'NONE',  ( -13.39934810366954210, 164.7282670150663080, 312.4024525391586735 ) ) ;
#3700=AXIS2_PLACEMENT_3D ( 'NONE', #14520, #2194, #16127 ) ;
#3703=VERTEX_POINT ( 'NONE', #846 ) ;
#3718=PRESENTATION_STYLE_ASSIGNMENT (( #7276 ) ) ;
#3721=CARTESIAN_POINT ( 'NONE',  ( 15.52111512002419502, 188.5491499182944608, 308.4788755532068194 ) ) ;
#3756=CARTESIAN_POINT ( 'NONE',  ( -11.04227196300320912, 183.6076801826763187, 320.9867185712774926 ) ) ;
#3766=CARTESIAN_POINT ( 'NONE',  ( -15.18603124401100679, 179.4839357967852607, 314.7101063110252426 ) ) ;
#3778=DIRECTION ( 'NONE',  ( 0.3102455404053333088, 0.9506564598521396459, 0.000000000000000000 ) ) ;
#3793=CARTESIAN_POINT ( 'NONE',  ( -5.563703806604332058, 326.7005119474492290, 320.3383740725300299 ) ) ;
#3804=DIRECTION ( 'NONE',  ( -0.01292394549866745720, -0.005513023399720816918, -0.9999012842304692006 ) ) ;
#3817=CARTESIAN_POINT ( 'NONE',  ( -23.03053847350000538, 324.7037969250150695, 320.5318774195161495 ) ) ;
#3826=TOROIDAL_SURFACE ( 'NONE', #20309, 25.26969600708473607, 3.000000000000000000 ) ;
#3834=ORIENTED_EDGE ( 'NONE', *, *, #17947, .F. ) ;
#3844=CARTESIAN_POINT ( 'NONE',  ( 19.21689716288775074, 184.4993076657424353, 311.6842248372922199 ) ) ;
#3871=CARTESIAN_POINT ( 'NONE',  ( -13.02223955641218822, 183.9466781734064114, 319.8591424033813837 ) ) ;
#3875=CARTESIAN_POINT ( 'NONE',  ( -5.860583941020064636, 326.6140704304781366, 307.3310200717714338 ) ) ;
#3876=CARTESIAN_POINT ( 'NONE',  ( -13.61876686344269416, 180.6360036619030893, 319.1235917264722275 ) ) ;
#3897=CARTESIAN_POINT ( 'NONE',  ( -8.515086503764345949, 185.4173453262823728, 305.3464451745876431 ) ) ;
#3917=CARTESIAN_POINT ( 'NONE',  ( -10.18122515959160701, 165.1294603137475860, 320.6223196198712913 ) ) ;
#3926=ORIENTED_EDGE ( 'NONE', *, *, #17629, .T. ) ;
#3928=CARTESIAN_POINT ( 'NONE',  ( 16.39634482804422433, 187.9401017119210451, 319.7988598509798521 ) ) ;
#3940=CARTESIAN_POINT ( 'NONE',  ( 18.61482433265386405, 185.2913030115592221, 310.7831755306406762 ) ) ;
#3953=VERTEX_POINT ( 'NONE', #8439 ) ;
#3958=CARTESIAN_POINT ( 'NONE',  ( 12.98486085753333263, 190.3233720689114818, 320.8552415163618434 ) ) ;
#3970=CARTESIAN_POINT ( 'NONE',  ( -15.08775915360043207, 178.5843476654970914, 314.2199384936897104 ) ) ;
#3977=CARTESIAN_POINT ( 'NONE',  ( 12.15711459821606155, 188.6915557983204224, 307.0876295708031876 ) ) ;
#3980=EDGE_LOOP ( 'NONE', ( #15650, #18663, #20093, #5836, #16555 ) ) ;
#3987=CARTESIAN_POINT ( 'NONE',  ( -13.92525281995234820, 325.7770340667113942, 328.4523304068723064 ) ) ;
#3998=COLOUR_RGB ( '', 0.72549020, 0.75294118, 0.79215686) ;
#3999=CARTESIAN_POINT ( 'NONE',  ( -3.030255530017816668, 323.0571258370100054, 414.2134192087003726 ) ) ;
#4020=VERTEX_POINT ( 'NONE', #14790 ) ;
#4044=ORIENTED_EDGE ( 'NONE', *, *, #4897, .T. ) ;
#4053=CARTESIAN_POINT ( 'NONE',  ( 20.55381086804826651, 182.0128392866518823, 312.7933888596797374 ) ) ;
#4057=SHAPE_REPRESENTATION_RELATIONSHIP ( 'NONE' , 'NONE' ,  #15037, #13490 ) ;
#4063=CARTESIAN_POINT ( 'NONE',  ( -10.02112475001242586, 187.8727749214653784, 308.1601357688390408 ) ) ;
#4081=CARTESIAN_POINT ( 'NONE',  ( -8.641754912934437982, 185.9330366646549066, 321.2360663095644213 ) ) ;
#4086=DIRECTION ( 'NONE',  ( -0.01292394549866745720, -0.005513023399720816918, -0.9999012842304692006 ) ) ;
#4087=VECTOR ( 'NONE', #1216, 1000.000000000000227 ) ;
#4089=ADVANCED_FACE ( 'NONE', ( #21512 ), #20480, .F. ) ;
#4091=CARTESIAN_POINT ( 'NONE',  ( -9.868119059700692475, 184.4438714364067380, 308.0446564981782558 ) ) ;
#4094=AXIS2_PLACEMENT_3D ( 'NONE', #12668, #3804, #249 ) ;
#4095=VERTEX_POINT ( 'NONE', #21847 ) ;
#4100=CIRCLE ( 'NONE', #5567, 20.50000000000000000 ) ;
#4110=CARTESIAN_POINT ( 'NONE',  ( 12.38356306630694803, 188.4816022558815973, 321.6789667137223319 ) ) ;
#4112=CARTESIAN_POINT ( 'NONE',  ( -9.622921994803601109, 336.0360340286487713, 414.2270707938455416 ) ) ;
#4135=VERTEX_POINT ( 'NONE', #11429 ) ;
#4142=CARTESIAN_POINT ( 'NONE',  ( -7.939077925311260664, 165.3359731837102515, 308.2574871822228033 ) ) ;
#4151=CARTESIAN_POINT ( 'NONE',  ( 12.82460312764358612, 190.4936219940274498, 307.8489606432475512 ) ) ;
#4172=CARTESIAN_POINT ( 'NONE',  ( 19.67111680476709168, 183.8698952613492281, 312.7070380754294661 ) ) ;
#4180=DIRECTION ( 'NONE',  ( 0.9935244165829104634, 0.1136188085379686713, 0.000000000000000000 ) ) ;
#4208=CARTESIAN_POINT ( 'NONE',  ( -11.50381294012838040, 186.2556874024963065, 308.5302510577426460 ) ) ;
#4213=CARTESIAN_POINT ( 'NONE',  ( 11.96358776207564567, 188.1236699898683185, 306.3470157435421015 ) ) ;
#4222=CARTESIAN_POINT ( 'NONE',  ( -12.34320795831280826, 182.0705588102794650, 322.4648799061273508 ) ) ;
#4230=FACE_OUTER_BOUND ( 'NONE', #22663, .T. ) ;
#4245=CARTESIAN_POINT ( 'NONE',  ( 3.943435745640934798, 166.6820924781355302, 305.0961849656022764 ) ) ;
#4263=CARTESIAN_POINT ( 'NONE',  ( 12.83416875720839911, 190.4899810681968972, 307.8495766059611469 ) ) ;
#4276=ORIENTED_EDGE ( 'NONE', *, *, #5816, .T. ) ;
#4279=CARTESIAN_POINT ( 'NONE',  ( 19.65679901206711477, 183.0231349956771112, 316.5272444403498184 ) ) ;
#4296=DIRECTION ( 'NONE',  ( -0.01292394549866745720, -0.005513023399720816918, -0.9999012842304692006 ) ) ;
#4305=CARTESIAN_POINT ( 'NONE',  ( -8.326885050334665195, 185.3762957732174073, 323.2536174830050868 ) ) ;
#4311=CARTESIAN_POINT ( 'NONE',  ( -12.22164657274376154, 182.3338479205205260, 308.9437607284932028 ) ) ;
#4319=TOROIDAL_SURFACE ( 'NONE', #6530, 17.29295143883736330, 7.000000000000003553 ) ;
#4325=ORIENTED_EDGE ( 'NONE', *, *, #11346, .F. ) ;
#4328=CARTESIAN_POINT ( 'NONE',  ( -15.37386863723000907, 178.0286960282952862, 316.7568799295810891 ) ) ;
#4334=ORIENTED_EDGE ( 'NONE', *, *, #20873, .F. ) ;
#4337=CARTESIAN_POINT ( 'NONE',  ( -8.832654921828126504, 186.0492927733070587, 307.0981779263103135 ) ) ;
#4385=CIRCLE ( 'NONE', #19066, 1.999999999999998224 ) ;
#4389=CARTESIAN_POINT ( 'NONE',  ( 17.35622542770311938, 184.9967961627334887, 319.5060476712728814 ) ) ;
#4405=CARTESIAN_POINT ( 'NONE',  ( -9.841028579513169561, 187.8130746588807938, 321.1594247271215750 ) ) ;
#4410=CIRCLE ( 'NONE', #2227, 25.26969600708473962 ) ;
#4429=CARTESIAN_POINT ( 'NONE',  ( -14.35744025451807104, 179.7190799334499332, 309.4176276921488125 ) ) ;
#4432=EDGE_LOOP ( 'NONE', ( #7899, #917, #11968, #20969 ) ) ;
#4450=CARTESIAN_POINT ( 'NONE',  ( -8.747090466623152594, 185.2634439126724999, 305.1792882774458917 ) ) ;
#4459=CARTESIAN_POINT ( 'NONE',  ( -26.20953091143350377, 324.3346178683207768, 319.1363590876133571 ) ) ;
#4469=CARTESIAN_POINT ( 'NONE',  ( 13.04687021101641342, 190.3009381008880609, 320.8498765639175190 ) ) ;
#4470=DIRECTION ( 'NONE',  ( -0.01292394549866727679, -0.005513023399720742325, -0.9999012842304692006 ) ) ;
#4481=DIRECTION ( 'NONE',  ( 0.01292394549866727679, 0.005513023399720742325, 0.9999012842304692006 ) ) ;
#4510=CARTESIAN_POINT ( 'NONE',  ( 19.89301572175062560, 183.5588582068999131, 313.6515632266070384 ) ) ;
#4521=ORIENTED_EDGE ( 'NONE', *, *, #7164, .F. ) ;
#4523=DIRECTION ( 'NONE',  ( 0.1136178953597579422, -0.9935164314186355483, 0.004009283626633659663 ) ) ;
#4542=AXIS2_PLACEMENT_3D ( 'NONE', #6910, #1648, #24 ) ;
#4546=CARTESIAN_POINT ( 'NONE',  ( -10.58768000256260855, 183.8591665011366842, 305.6983654296078043 ) ) ;
#4554=CARTESIAN_POINT ( 'NONE',  ( 0.3024632767450905479, 327.3415402339139746, 312.9481704872475234 ) ) ;
#4561=CARTESIAN_POINT ( 'NONE',  ( -15.56327362081419885, 177.7277181364938485, 314.9118054635637236 ) ) ;
#4583=DIRECTION ( 'NONE',  ( -0.9934404589540164476, -0.1135548637187044213, 0.01346653032743048289 ) ) ;
#4587=B_SPLINE_SURFACE_WITH_KNOTS ( 'NONE', 3, 1, ( 
 ( #3875, #19375 ),
 ( #17562, #1813 ),
 ( #7091, #14123 ),
 ( #1934, #210 ),
 ( #7206, #14237 ),
 ( #21212, #5467 ),
 ( #12504, #19490 ),
 ( #16081, #322 ),
 ( #7313, #21325 ),
 ( #5593, #12628 ),
 ( #15763, #14040 ),
 ( #5158, #10467 ),
 ( #16106, #6887 ),
 ( #17483, #22596 ),
 ( #6, #19182 ),
 ( #21022, #13910 ),
 ( #350, #21236 ),
 ( #1734, #19065 ),
 ( #128, #12200 ),
 ( #5501, #239 ),
 ( #12532, #20901 ),
 ( #8955, #7233 ),
 ( #12319, #16000 ),
 ( #7128, #7009 ),
 ( #5275, #17719 ),
 ( #8610, #7342 ),
 ( #3669, #3454 ),
 ( #8711, #15652 ),
 ( #19296, #1965 ),
 ( #14263, #3560 ),
 ( #10572, #17594 ),
 ( #3336, #19526 ),
 ( #3793, #14156 ),
 ( #10815, #21135 ),
 ( #10358, #1840 ),
 ( #8838, #5381 ) ),
 .UNSPECIFIED., .F., .F., .F.,
 ( 4, 3, 2, 2, 2, 2, 2, 2, 2, 2, 2, 2, 2, 2, 2, 3, 4 ),
 ( 2, 2 ),
 ( -0.01000000000000000021, 0.000000000000000000, 0.1249999999999998335, 0.1874999999999999167, 0.2500000000000000000, 0.3125000000000000555, 0.3750000000000001665, 0.4375000000000002220, 0.5000000000000003331, 0.5625000000000003331, 0.6250000000000003331, 0.6875000000000004441, 0.7500000000000004441, 0.8125000000000004441, 0.8750000000000004441, 1.000000000000000000, 1.010000000000000009 ),
 ( 0.000000000000000000, 1.000000000000000000 ),
 .UNSPECIFIED. ) ;
#4616=ORIENTED_EDGE ( 'NONE', *, *, #6425, .F. ) ;
#4631=CARTESIAN_POINT ( 'NONE',  ( -10.47529108877129289, 187.0770174862624629, 321.0793257476343570 ) ) ;
#4651=CARTESIAN_POINT ( 'NONE',  ( -8.455960479418571651, 185.4572466408051241, 305.1464658859009660 ) ) ;
#4660=CARTESIAN_POINT ( 'NONE',  ( -11.71580855312696201, 182.8374334212718395, 306.3219252926489276 ) ) ;
#4662=CARTESIAN_POINT ( 'NONE',  ( 16.39634482804422433, 187.9401017119210451, 319.7988598509798521 ) ) ;
#4671=CARTESIAN_POINT ( 'NONE',  ( -27.41563077536688908, 324.1610551366917434, 310.3061288224688496 ) ) ;
#4680=DIRECTION ( 'NONE',  ( -0.01292394549866727679, -0.005513023399720742325, -0.9999012842304692006 ) ) ;
#4686=EDGE_CURVE ( 'NONE', #5262, #19478, #1802, .T. ) ;
#4713=ORIENTED_EDGE ( 'NONE', *, *, #5675, .T. ) ;
#4715=AXIS2_PLACEMENT_3D ( 'NONE', #11818, #13536, #15279 ) ;
#4733=ORIENTED_EDGE ( 'NONE', *, *, #18206, .T. ) ;
#4735=VERTEX_POINT ( 'NONE', #3234 ) ;
#4748=LINE ( 'NONE', #20612, #9569 ) ;
#4768=CARTESIAN_POINT ( 'NONE',  ( -4.135966696445571245, 326.8123805703096423, 307.5996468166270006 ) ) ;
#4769=CARTESIAN_POINT ( 'NONE',  ( -9.829263477007989636, 187.6861072963453125, 321.1599754959502775 ) ) ;
#4771=CARTESIAN_POINT ( 'NONE',  ( 15.78165906541865304, 186.0656686932232446, 322.5043251233448700 ) ) ;
#4785=DIRECTION ( 'NONE',  ( -0.01292394549866745720, -0.005513023399720816918, -0.9999012842304692006 ) ) ;
#4788=CARTESIAN_POINT ( 'NONE',  ( -12.82378010018955550, 184.2676410047889703, 320.0244981536045543 ) ) ;
#4884=ADVANCED_FACE ( 'NONE', ( #13430, #20640 ), #17320, .F. ) ;
#4888=EDGE_CURVE ( 'NONE', #17417, #17190, #17975, .T. ) ;
#4893=DIRECTION ( 'NONE',  ( 0.3101392564284309317, 0.9506461370142480494, -0.009250070373105347826 ) ) ;
#4896=AXIS2_PLACEMENT_3D ( 'NONE', #2983, #10001, #17027 ) ;
#4897=EDGE_CURVE ( 'NONE', #1183, #1264, #12473, .T. ) ;
#4905=PLANE ( 'NONE',  #18049 ) ;
#4907=PLANE ( 'NONE',  #14706 ) ;
#4909=CARTESIAN_POINT ( 'NONE',  ( -11.71322822773759320, 182.7629020050958673, 320.7064967533905246 ) ) ;
#4951=ORIENTED_EDGE ( 'NONE', *, *, #22283, .F. ) ;
#4967=ADVANCED_FACE ( 'NONE', ( #20854 ), #8244, .F. ) ;
#4974=AXIS2_PLACEMENT_3D ( 'NONE', #10223, #6873, #13791 ) ;
#4988=CARTESIAN_POINT ( 'NONE',  ( -8.689953299324470137, 185.3004383898032188, 305.1731502674360286 ) ) ;
#4995=CARTESIAN_POINT ( 'NONE',  ( 13.02962957137955335, 190.4272972286120478, 320.8494027134000817 ) ) ;
#4997=( BOUNDED_SURFACE ( )  B_SPLINE_SURFACE ( 3, 2, ( 
 ( #1376, #22237, #6529 ),
 ( #20524, #4909, #4788 ),
 ( #11940, #18926, #10205 ),
 ( #14356, #3640, #9029 ),
 ( #211, #9148, #19818 ),
 ( #21326, #5469, #21213 ),
 ( #12734, #3876, #16199 ),
 ( #12505, #1935, #7314 ),
 ( #15854, #5357, #17914 ),
 ( #12397, #14238, #8925 ),
 ( #7207, #12842, #10544 ),
 ( #10993, #323, #10887 ),
 ( #17563, #2148, #15972 ),
 ( #21101, #7437, #16082 ),
 ( #5594, #17810, #19491 ),
 ( #12629, #19376, #7555 ),
 ( #19701, #2044, #1814 ),
 ( #14477, #21442, #439 ),
 ( #8800, #5702, #3766 ),
 ( #10654, #3970, #19603 ),
 ( #18023, #2271, #10778 ),
 ( #9270, #16317, #557 ),
 ( #97, #14582, #21538 ),
 ( #5808, #7093, #14124 ),
 ( #17689, #11236, #9384 ),
 ( #18241, #21987, #14695 ),
 ( #18340, #7778, #9624 ),
 ( #15153, #21763, #9841 ),
 ( #11459, #13087, #21647 ),
 ( #16861, #11574, #5936 ),
 ( #4429, #14932, #20054 ),
 ( #6404, #16652, #16759 ),
 ( #2394, #16421, #6288 ),
 ( #18466, #902, #1125 ),
 ( #2731, #13313, #9744 ),
 ( #18573, #2496, #8120 ),
 ( #20283, #4311, #7995 ),
 ( #9495, #1007, #2834 ),
 ( #15033, #11340, #13422 ),
 ( #4546, #16530, #4208 ),
 ( #22102, #4091, #7892 ),
 ( #11123, #21871, #18143 ),
 ( #664, #12973, #7652 ),
 ( #19938, #782, #14815 ),
 ( #6058, #2613, #6168 ),
 ( #13193, #20161, #15267 ),
 ( #3396, #22216, #1352 ),
 ( #4988, #17091, #22644 ),
 ( #20392, #11682, #3159 ),
 ( #8553, #16986, #10408 ),
 ( #15594, #18797, #13752 ),
 ( #12016, #8329, #6940 ),
 ( #4651, #18673, #10178 ),
 ( #8658, #15702, #1247 ) ),
 .UNSPECIFIED., .F., .F., .T. ) 
 B_SPLINE_SURFACE_WITH_KNOTS ( ( 4, 2, 2, 2, 2, 2, 2, 2, 2, 2, 2, 2, 2, 2, 2, 2, 2, 2, 2, 2, 2, 2, 2, 2, 2, 2, 4 ),
 ( 3, 3 ),
 ( 0.1301284894805934678, 0.1318527056069465075, 0.1335769217332995473, 0.1353011378596525871, 0.1361632459228291070, 0.1370253539860056269, 0.1387495701123586667, 0.1396116781755351866, 0.1404737862387117064, 0.1413358943018882263, 0.1421980023650647462, 0.1430601104282412661, 0.1439222184914177860, 0.1456464346177708258, 0.1465085426809473457, 0.1473706507441238656, 0.1490948668704769053, 0.1499569749336534252, 0.1508190829968299451, 0.1542675152495360247, 0.1551296233127125446, 0.1559917313758890645, 0.1568538394390656121, 0.1572848934706538859, 0.1573926569785509544, 0.1575004204864480228, 0.1577159475022421320 ),
 ( 0.000000000000000000, 1.000000000000000000 ),
 .UNSPECIFIED. ) 
 GEOMETRIC_REPRESENTATION_ITEM ( )  RATIONAL_B_SPLINE_SURFACE ( (
 ( 1.000000000000000000, 0.8227386401542207128, 1.000000000000000000),
 ( 1.000000000000000000, 0.8333712125770807999, 1.000000000000000000),
 ( 1.000000000000000000, 0.8437848470051855232, 1.000000000000000000),
 ( 1.000000000000000000, 0.8640507908242766044, 1.000000000000000000),
 ( 1.000000000000000000, 0.8738632290070461606, 1.000000000000000000),
 ( 1.000000000000000000, 0.8923321234614439712, 1.000000000000000000),
 ( 1.000000000000000000, 0.9010134951843085105, 1.000000000000000000),
 ( 1.000000000000000000, 0.9129850007871143092, 1.000000000000000000),
 ( 1.000000000000000000, 0.9168115705809977145, 1.000000000000000000),
 ( 1.000000000000000000, 0.9241129455457998132, 1.000000000000000000),
 ( 1.000000000000000000, 0.9275997298644027556, 1.000000000000000000),
 ( 1.000000000000000000, 0.9371813536878720319, 1.000000000000000000),
 ( 1.000000000000000000, 0.9425342029318131143, 1.000000000000000000),
 ( 1.000000000000000000, 0.9487217190514500853, 1.000000000000000000),
 ( 1.000000000000000000, 0.9504219373548455918, 1.000000000000000000),
 ( 1.000000000000000000, 0.9530138574316157074, 1.000000000000000000),
 ( 1.000000000000000000, 0.9539189288212627238, 1.000000000000000000),
 ( 1.000000000000000000, 0.9548931618690527090, 1.000000000000000000),
 ( 1.000000000000000000, 0.9549507483037429356, 1.000000000000000000),
 ( 1.000000000000000000, 0.9541752437097101858, 1.000000000000000000),
 ( 1.000000000000000000, 0.9533611900843690368, 1.000000000000000000),
 ( 1.000000000000000000, 0.9509603907209587259, 1.000000000000000000),
 ( 1.000000000000000000, 0.9493731739221451527, 1.000000000000000000),
 ( 1.000000000000000000, 0.9454412650859107536, 1.000000000000000000),
 ( 1.000000000000000000, 0.9431063129023899982, 1.000000000000000000),
 ( 1.000000000000000000, 0.9353430921237518847, 1.000000000000000000),
 ( 1.000000000000000000, 0.9290748369521870664, 1.000000000000000000),
 ( 1.000000000000000000, 0.9182885162027015769, 1.000000000000000000),
 ( 1.000000000000000000, 0.9144642180539555021, 1.000000000000000000),
 ( 1.000000000000000000, 0.9065214887599388760, 1.000000000000000000),
 ( 1.000000000000000000, 0.9023952855941976825, 1.000000000000000000),
 ( 1.000000000000000000, 0.8895549064154443242, 1.000000000000000000),
 ( 1.000000000000000000, 0.8803896720082297067, 1.000000000000000000),
 ( 1.000000000000000000, 0.8659833981722644403, 1.000000000000000000),
 ( 1.000000000000000000, 0.8610623523000291435, 1.000000000000000000),
 ( 1.000000000000000000, 0.8509715058880433780, 1.000000000000000000),
 ( 1.000000000000000000, 0.8457963385677346180, 1.000000000000000000),
 ( 1.000000000000000000, 0.8197273272024717672, 1.000000000000000000),
 ( 1.000000000000000000, 0.7979877476287833282, 1.000000000000000000),
 ( 1.000000000000000000, 0.7710357334748190183, 1.000000000000000000),
 ( 1.000000000000000000, 0.7656985913657583520, 1.000000000000000000),
 ( 1.000000000000000000, 0.7550404585215626518, 1.000000000000000000),
 ( 1.000000000000000000, 0.7497880368474888479, 1.000000000000000000),
 ( 1.000000000000000000, 0.7395325035323125906, 1.000000000000000000),
 ( 1.000000000000000000, 0.7345293846932524628, 1.000000000000000000),
 ( 1.000000000000000000, 0.7272879817929819302, 1.000000000000000000),
 ( 1.000000000000000000, 0.7249181014104938425, 1.000000000000000000),
 ( 1.000000000000000000, 0.7220190359316460693, 1.000000000000000000),
 ( 1.000000000000000000, 0.7214423886269636377, 1.000000000000000000),
 ( 1.000000000000000000, 0.7202956422195359032, 1.000000000000000000),
 ( 1.000000000000000000, 0.7204858121524565506, 1.000000000000000000),
 ( 1.000000000000000000, 0.7203839998076618789, 1.000000000000000000),
 ( 1.000000000000000000, 0.7203159680551509680, 1.000000000000000000),
 ( 1.000000000000000000, 0.7202477793832563480, 1.000000000000000000) ) ) 
 REPRESENTATION_ITEM ( '' )  SURFACE ( )  );
#5002=CARTESIAN_POINT ( 'NONE',  ( 12.52469039290287611, 187.5804275016522240, 322.9582397512710941 ) ) ;
#5006=DIRECTION ( 'NONE',  ( 0.9934404589540153374, 0.1135548637187135251, -0.01346653032743037014 ) ) ;
#5007=EDGE_CURVE ( 'NONE', #1264, #1183, #20129, .T. ) ;
#5010=VERTEX_POINT ( 'NONE', #308 ) ;
#5015=CARTESIAN_POINT ( 'NONE',  ( 16.38239381841655984, 185.4577457402829168, 306.4392643500532927 ) ) ;
#5020=EDGE_CURVE ( 'NONE', #7715, #5612, #18454, .T. ) ;
#5039=ORIENTED_EDGE ( 'NONE', *, *, #22361, .F. ) ;
#5041=CARTESIAN_POINT ( 'NONE',  ( -3.975234144917287438, 326.8809449508823946, 320.0352211315558293 ) ) ;
#5079=B_SPLINE_CURVE_WITH_KNOTS ( 'NONE', 3,
 ( #4469, #13347, #22249, #9664, #18832, #16692, #9773, #7926, #20425, #6088, #13556, #17021, #6201, #16895, #13228 ),
 .UNSPECIFIED., .F., .F.,
 ( 4, 2, 1, 1, 1, 2, 2, 2, 4 ),
 ( -5.999999999001200712E-08, 3.336925554464112399E-05, 6.679851108927226935E-05, 0.0001336570221785711248, 0.0002673740443571829845, 0.0005348080887144481205, 0.001069676177429040734, 0.002139412354858207313, 0.004278884709716497536 ),
 .UNSPECIFIED. ) ;
#5100=ORIENTED_EDGE ( 'NONE', *, *, #19412, .T. ) ;
#5103=AXIS2_PLACEMENT_3D ( 'NONE', #3987, #2287, #1140 ) ;
#5110=AXIS2_PLACEMENT_3D ( 'NONE', #11239, #17916, #2152 ) ;
#5111=CARTESIAN_POINT ( 'NONE',  ( 16.40873467034997191, 185.6567299720572350, 322.3321779654821171 ) ) ;
#5131=EDGE_LOOP ( 'NONE', ( #15559, #18865, #15546, #21097 ) ) ;
#5140=DIRECTION ( 'NONE',  ( -0.01292394549866727679, -0.005513023399720743192, -0.9999012842304693116 ) ) ;
#5158=CARTESIAN_POINT ( 'NONE',  ( -1.405147466491028840, 327.1319313373589353, 309.3977247008179461 ) ) ;
#5165=DIRECTION ( 'NONE',  ( 0.9934404589540163366, 0.1135548637187057258, -0.01346653032743021922 ) ) ;
#5168=EDGE_CURVE ( 'NONE', #8739, #9852, #17292, .T. ) ;
#5176=ORIENTED_EDGE ( 'NONE', *, *, #4888, .T. ) ;
#5181=CARTESIAN_POINT ( 'NONE',  ( -23.62788402525385578, 324.6350553711861835, 320.4254447255032119 ) ) ;
#5188=CIRCLE ( 'NONE', #8867, 22.50000000000000355 ) ;
#5196=CARTESIAN_POINT ( 'NONE',  ( 19.33710169866840189, 184.3365238270897066, 311.8886436260900723 ) ) ;
#5211=CARTESIAN_POINT ( 'NONE',  ( 12.02049240483441750, 187.6813724364916425, 304.8898053572733602 ) ) ;
#5228=CARTESIAN_POINT ( 'NONE',  ( 13.12964460975451608, 190.2538275423460163, 320.8426553563187440 ) ) ;
#5229=VERTEX_POINT ( 'NONE', #8426 ) ;
#5232=CARTESIAN_POINT ( 'NONE',  ( -11.02481633791520998, 186.5310056599434176, 320.9512889225665049 ) ) ;
#5243=CARTESIAN_POINT ( 'NONE',  ( 19.98044029014978307, 182.5758476881784702, 310.8270597400842234 ) ) ;
#5262=VERTEX_POINT ( 'NONE', #5985 ) ;
#5275=CARTESIAN_POINT ( 'NONE',  ( -1.291844632700186013, 327.1802634178375797, 318.1637512231440041 ) ) ;
#5299=CARTESIAN_POINT ( 'NONE',  ( -22.40767239932358379, 324.7751959534260777, 320.5736243973683486 ) ) ;
#5314=CARTESIAN_POINT ( 'NONE',  ( 19.91562502177398386, 183.5286201153226386, 313.8266703284822938 ) ) ;
#5325=CARTESIAN_POINT ( 'NONE',  ( 11.99112089040652762, 187.7242859511004838, 307.7456636232291203 ) ) ;
#5334=VERTEX_POINT ( 'NONE', #7706 ) ;
#5346=ORIENTED_EDGE ( 'NONE', *, *, #637, .T. ) ;
#5349=FACE_OUTER_BOUND ( 'NONE', #10093, .T. ) ;
#5353=CARTESIAN_POINT ( 'NONE',  ( -13.60878576479588276, 182.9261561738083515, 319.2680663699061370 ) ) ;
#5357=CARTESIAN_POINT ( 'NONE',  ( -14.05315427626016600, 180.0651354203414769, 318.4885795860537314 ) ) ;
#5359=CARTESIAN_POINT ( 'NONE',  ( 16.60281234097334746, 185.5290831433204062, 322.2010377526273146 ) ) ;
#5364=CARTESIAN_POINT ( 'NONE',  ( 24.56098209142228228, 169.1174711406635822, 324.3181961363840742 ) ) ;
#5377=LINE ( 'NONE', #3662, #15862 ) ;
#5381=CARTESIAN_POINT ( 'NONE',  ( 15.94290392677929269, 168.1183014920872267, 320.9451345667529836 ) ) ;
#5393=TOROIDAL_SURFACE ( 'NONE', #1399, 17.29295143883736330, 7.000000000000003553 ) ;
#5403=CARTESIAN_POINT ( 'NONE',  ( -12.21093709921540338, 164.8562217133218439, 310.4321100316089428 ) ) ;
#5423=ORIENTED_EDGE ( 'NONE', *, *, #5863, .F. ) ;
#5434=CARTESIAN_POINT ( 'NONE',  ( 13.02529137814181048, 190.3775507350028136, 307.8631787466416085 ) ) ;
#5454=CARTESIAN_POINT ( 'NONE',  ( 12.32651890270660644, 188.3103955803847782, 320.9483625192488034 ) ) ;
#5458=LINE ( 'NONE', #15842, #9540 ) ;
#5467=CARTESIAN_POINT ( 'NONE',  ( 17.03779215356004073, 168.1915823533492755, 308.0767119223879718 ) ) ;
#5469=CARTESIAN_POINT ( 'NONE',  ( -13.37948476813407872, 180.9346274286824325, 319.4053979151471481 ) ) ;
#5470=CARTESIAN_POINT ( 'NONE',  ( 20.68288668254167462, 181.8935073550437664, 313.8768750210967369 ) ) ;
#5484=VERTEX_POINT ( 'NONE', #19836 ) ;
#5501=CARTESIAN_POINT ( 'NONE',  ( 0.2676632691968778843, 327.3448798950369110, 314.7619388544391654 ) ) ;
#5524=CARTESIAN_POINT ( 'NONE',  ( -12.75205171465932352, 164.7972115514004088, 311.1436431959231754 ) ) ;
#5540=UNCERTAINTY_MEASURE_WITH_UNIT (LENGTH_MEASURE( 1.000000000000000082E-05 ), #14086, 'distance_accuracy_value', 'NONE');
#5556=CARTESIAN_POINT ( 'NONE',  ( 19.01596917749679250, 183.5201396444011266, 310.9998942482669690 ) ) ;
#5561=CARTESIAN_POINT ( 'NONE',  ( -8.750674252510810547, 186.0658606611824553, 321.9654507654339000 ) ) ;
#5567=AXIS2_PLACEMENT_3D ( 'NONE', #10893, #16658, #565 ) ;
#5579=CARTESIAN_POINT ( 'NONE',  ( 12.18842727924546665, 188.3644011796234565, 320.9609158465759720 ) ) ;
#5593=CARTESIAN_POINT ( 'NONE',  ( -2.342497703613107607, 327.0213694383911047, 308.5633357006506117 ) ) ;
#5594=CARTESIAN_POINT ( 'NONE',  ( -15.43087866951515608, 177.9355826206890470, 316.4028962195858981 ) ) ;
#5606=ORIENTED_EDGE ( 'NONE', *, *, #22283, .T. ) ;
#5612=VERTEX_POINT ( 'NONE', #14375 ) ;
#5615=CARTESIAN_POINT ( 'NONE',  ( 12.81118841006561304, 189.7386529835138731, 320.9279672944379058 ) ) ;
#5624=ADVANCED_FACE ( 'NONE', ( #19619 ), #2186, .F. ) ;
#5643=AXIS2_PLACEMENT_3D ( 'NONE', #11511, #15529, #8946 ) ;
#5645=CARTESIAN_POINT ( 'NONE',  ( -7.728110352850903197, 165.4125665588315144, 321.2590829791397482 ) ) ;
#5666=CARTESIAN_POINT ( 'NONE',  ( 11.87914702380516019, 187.7661313520924296, 307.7599159327405687 ) ) ;
#5675=EDGE_CURVE ( 'NONE', #1967, #17055, #21882, .T. ) ;
#5678=ORIENTED_EDGE ( 'NONE', *, *, #8353, .T. ) ;
#5689=CARTESIAN_POINT ( 'NONE',  ( 12.27027136777087790, 187.6773065828753602, 322.9709648702423692 ) ) ;
#5691=EDGE_LOOP ( 'NONE', ( #10486, #5346, #20115, #1205 ) ) ;
#5696=CARTESIAN_POINT ( 'NONE',  ( -8.650559030193861076, 185.1599980327158335, 323.2452797403996101 ) ) ;
#5700=CARTESIAN_POINT ( 'NONE',  ( -14.48915200586460372, 181.2968306206680325, 311.4287039645396931 ) ) ;
#5702=CARTESIAN_POINT ( 'NONE',  ( -15.10148691740612747, 178.5546173124768927, 314.7004641218159691 ) ) ;
#5771=CARTESIAN_POINT ( 'NONE',  ( 17.89548223907189950, 186.1632423467296462, 310.0097253882542532 ) ) ;
#5778=CARTESIAN_POINT ( 'NONE',  ( -10.02115732914335489, 187.8727529749444045, 308.1601390762862138 ) ) ;
#5808=CARTESIAN_POINT ( 'NONE',  ( -15.36585396882763277, 178.1140882805800345, 312.4503017070314286 ) ) ;
#5811=VERTEX_POINT ( 'NONE', #20859 ) ;
#5814=ORIENTED_EDGE ( 'NONE', *, *, #8533, .F. ) ;
#5816=EDGE_CURVE ( 'NONE', #18739, #20005, #16886, .T. ) ;
#5832=CARTESIAN_POINT ( 'NONE',  ( 12.41900304340602368, 188.5914010946799806, 321.5742196380866744 ) ) ;
#5836=ORIENTED_EDGE ( 'NONE', *, *, #27, .F. ) ;
#5853=DIRECTION ( 'NONE',  ( 0.01292394549866741557, 0.005513023399720776152, 0.9999012842304692006 ) ) ;
#5863=EDGE_CURVE ( 'NONE', #11287, #6191, #5458, .T. ) ;
#5874=ORIENTED_EDGE ( 'NONE', *, *, #21827, .T. ) ;
#5887=ORIENTED_EDGE ( 'NONE', *, *, #14435, .T. ) ;
#5897=CARTESIAN_POINT ( 'NONE',  ( 20.06961194383113067, 182.5783991459622655, 314.4765814583797123 ) ) ;
#5926=CARTESIAN_POINT ( 'NONE',  ( -8.413499874523651556, 185.3190104300268217, 323.2517229709724234 ) ) ;
#5936=CARTESIAN_POINT ( 'NONE',  ( -14.38384282170848572, 181.5288438622440026, 311.2293654625956947 ) ) ;
#5942=CARTESIAN_POINT ( 'NONE',  ( 12.81503532323078964, 190.4972571607467842, 307.8483445055002221 ) ) ;
#5951=CARTESIAN_POINT ( 'NONE',  ( -15.09567095940728798, 178.4792087098117577, 317.9922241412446056 ) ) ;
#5954=ORIENTED_EDGE ( 'NONE', *, *, #14587, .F. ) ;
#5957=CARTESIAN_POINT ( 'NONE',  ( 12.32031054571417705, 188.2809068403609558, 321.9016682987510762 ) ) ;
#5960=ORIENTED_EDGE ( 'NONE', *, *, #14435, .F. ) ;
#5977=DIRECTION ( 'NONE',  ( -0.9934404589540163366, -0.1135548637187060866, 0.01346653032743036840 ) ) ;
#5985=CARTESIAN_POINT ( 'NONE',  ( -18.45420839006976621, 164.1078124625656187, 301.8995274031627787 ) ) ;
#6000=EDGE_LOOP ( 'NONE', ( #18341, #4334, #7973, #5039, #4616, #5960 ) ) ;
#6009=ORIENTED_EDGE ( 'NONE', *, *, #14081, .F. ) ;
#6016=CARTESIAN_POINT ( 'NONE',  ( -44.99638338670928306, 229.0513208305363548, 372.9597790112123334 ) ) ;
#6018=CARTESIAN_POINT ( 'NONE',  ( 20.00631865610750637, 182.6246599348329767, 313.5209380637898562 ) ) ;
#6025=( NAMED_UNIT ( * ) SI_UNIT ( $, .STERADIAN. ) SOLID_ANGLE_UNIT ( ) );
#6032=ORIENTED_EDGE ( 'NONE', *, *, #3400, .F. ) ;
#6042=CARTESIAN_POINT ( 'NONE',  ( 26.25061226286096883, 169.2177813299073819, 301.2935335384283917 ) ) ;
#6046=ORIENTED_EDGE ( 'NONE', *, *, #4686, .F. ) ;
#6058=CARTESIAN_POINT ( 'NONE',  ( -9.227205039120967456, 184.9256890989761644, 305.2585128821986018 ) ) ;
#6068=CARTESIAN_POINT ( 'NONE',  ( -13.49256607648177209, 180.7387789766418962, 321.2375318158862001 ) ) ;
#6080=CARTESIAN_POINT ( 'NONE',  ( -8.628845071887251805, 185.6862342536340691, 306.4543981107967738 ) ) ;
#6088=CARTESIAN_POINT ( 'NONE',  ( 13.81123123916535356, 189.8530796209156790, 320.7501109915356210 ) ) ;
#6089=FACE_OUTER_BOUND ( 'NONE', #10271, .T. ) ;
#6104=DIRECTION ( 'NONE',  ( -0.7480173694308205334, 0.4911576187806371285, 0.4463565934805150959 ) ) ;
#6128=CARTESIAN_POINT ( 'NONE',  ( 18.54778899613519982, 185.5359755103985719, 318.0241678234317533 ) ) ;
#6161=CARTESIAN_POINT ( 'NONE',  ( -8.391866834692953248, 185.3333697219060809, 323.2521960560945331 ) ) ;
#6163=ORIENTED_EDGE ( 'NONE', *, *, #16295, .F. ) ;
#6166=EDGE_LOOP ( 'NONE', ( #6328, #1798, #382, #22076, #1661, #21171 ) ) ;
#6168=CARTESIAN_POINT ( 'NONE',  ( -10.47940244875819538, 187.4174437848855348, 308.2255844705966297 ) ) ;
#6177=CARTESIAN_POINT ( 'NONE',  ( -5.731715098087014404, 326.6288426432528240, 307.3396573775339107 ) ) ;
#6180=PLANE ( 'NONE',  #22243 ) ;
#6182=CARTESIAN_POINT ( 'NONE',  ( -14.60065500149918805, 179.2330876351038285, 319.3326537707700936 ) ) ;
#6191=VERTEX_POINT ( 'NONE', #871 ) ;
#6201=CARTESIAN_POINT ( 'NONE',  ( 15.39737658676448895, 188.8107569276171773, 320.3072530890422627 ) ) ;
#6204=ORIENTED_EDGE ( 'NONE', *, *, #21833, .F. ) ;
#6212=CLOSED_SHELL ( 'NONE', ( #11995, #1634, #21656, #12256, #1822, #21563, #18897, #18492, #21796, #21789, #21879, #21815, #4884, #3064, #21276, #8373, #21868, #17240, #18245, #13908, #6795, #975, #10243, #17114, #15901, #13979, #4089, #4967, #1001, #18360, #21420, #5624, #17444, #19324 ) ) ;
#6231=TOROIDAL_SURFACE ( 'NONE', #2188, -102.0000000000000000, 120.0000000000000000 ) ;
#6240=AXIS2_PLACEMENT_3D ( 'NONE', #20523, #4785, #19031 ) ;
#6243=CARTESIAN_POINT ( 'NONE',  ( 19.73688183432247811, 182.9419304313151429, 316.3130507777162279 ) ) ;
#6270=CARTESIAN_POINT ( 'NONE',  ( 12.84378735233264379, 190.4863133572641232, 307.8501959441126701 ) ) ;
#6288=CARTESIAN_POINT ( 'NONE',  ( -13.90420332777824441, 182.5345320759501249, 310.4363584572501509 ) ) ;
#6292=AXIS2_PLACEMENT_3D ( 'NONE', #3102, #12069, #1395 ) ;
#6298=DIRECTION ( 'NONE',  ( 0.1136178953597579422, -0.9935164314186355483, 0.004009283626633659663 ) ) ;
#6301=CARTESIAN_POINT ( 'NONE',  ( 11.97603105386089872, 187.6983616241384709, 304.8864109523329375 ) ) ;
#6303=CARTESIAN_POINT ( 'NONE',  ( -15.37900450013992604, 178.0904888174965492, 312.5271116413751997 ) ) ;
#6308=CARTESIAN_POINT ( 'NONE',  ( -7.374421360215808186, 323.5613325621246190, 320.3790860758305712 ) ) ;
#6316=UNCERTAINTY_MEASURE_WITH_UNIT (LENGTH_MEASURE( 1.000000000000000082E-05 ), #10965, 'distance_accuracy_value', 'NONE');
#6328=ORIENTED_EDGE ( 'NONE', *, *, #7731, .F. ) ;
#6361=DIRECTION ( 'NONE',  ( 0.01292394549866727679, 0.005513023399720742325, 0.9999012842304692006 ) ) ;
#6368=CARTESIAN_POINT ( 'NONE',  ( 19.84368754553128866, 183.6791006555748424, 315.4184450387429592 ) ) ;
#6371=B_SPLINE_CURVE_WITH_KNOTS ( 'NONE', 3,
 ( #2522, #3897, #10915, #9525, #810, #6080, #7809, #21790, #4337, #9866, #11490, #22238, #14950, #18594, #21896, #16888, #13337, #22011 ),
 .UNSPECIFIED., .F., .F.,
 ( 4, 2, 2, 2, 2, 2, 2, 2, 4 ),
 ( -3.889482229076588469E-05, 0.0005389813425374914355, 0.001116857507365748769, 0.001694733672194006103, 0.002272609837022263653, 0.002850486001850521204, 0.003428362166678778321, 0.004006238331507035004, 0.004584114496335292555 ),
 .UNSPECIFIED. ) ;
#6393=DIRECTION ( 'NONE',  ( -0.01292394549866745720, -0.005513023399720816918, -0.9999012842304692006 ) ) ;
#6404=CARTESIAN_POINT ( 'NONE',  ( -14.03868214994468211, 180.1681535970077164, 308.8297336107179376 ) ) ;
#6425=EDGE_CURVE ( 'NONE', #19042, #15351, #4410, .T. ) ;
#6434=CARTESIAN_POINT ( 'NONE',  ( -23.46300067765492514, 324.6023353951521813, 307.6447243945494279 ) ) ;
#6435=EDGE_LOOP ( 'NONE', ( #22362, #1224, #14750, #6163 ) ) ;
#6442=VERTEX_POINT ( 'NONE', #7036 ) ;
#6483=ORIENTED_EDGE ( 'NONE', *, *, #9973, .T. ) ;
#6486=CARTESIAN_POINT ( 'NONE',  ( -11.79663605375380975, 185.7023549694303313, 320.6758801748541714 ) ) ;
#6518=CARTESIAN_POINT ( 'NONE',  ( 14.61723280919641255, 187.0110612265052339, 320.7690430450153372 ) ) ;
#6529=CARTESIAN_POINT ( 'NONE',  ( -12.58664483627160990, 184.6272112293441694, 320.1917372557447834 ) ) ;
#6530=AXIS2_PLACEMENT_3D ( 'NONE', #15952, #14103, #10631 ) ;
#6558=AXIS2_PLACEMENT_3D ( 'NONE', #16836, #20128, #16499 ) ;
#6580=CARTESIAN_POINT ( 'NONE',  ( 16.70266120485480243, 187.6440219821165840, 319.6249571544858554 ) ) ;
#6596=CARTESIAN_POINT ( 'NONE',  ( -12.01575389183062192, 182.4076787623453129, 322.7174846376778987 ) ) ;
#6601=CARTESIAN_POINT ( 'NONE',  ( 13.03496960693103546, 190.3881593399657390, 320.8495494816559130 ) ) ;
#6629=CARTESIAN_POINT ( 'NONE',  ( 13.46024906002343968, 187.7400488015692588, 320.9343290008155805 ) ) ;
#6638=DIRECTION ( 'NONE',  ( 0.9934404589540163366, 0.1135548637187057675, -0.01346653032742958604 ) ) ;
#6660=AXIS2_PLACEMENT_3D ( 'NONE', #10952, #19896, #2219 ) ;
#6678=VERTEX_POINT ( 'NONE', #12780 ) ;
#6726=EDGE_CURVE ( 'NONE', #1967, #15431, #15054, .T. ) ;
#6741=CARTESIAN_POINT ( 'NONE',  ( 12.61148133605082222, 188.1786184505010056, 320.9582656092828188 ) ) ;
#6744=FACE_OUTER_BOUND ( 'NONE', #11586, .T. ) ;
#6748=CARTESIAN_POINT ( 'NONE',  ( -18.15695764360042119, 164.2346120007591992, 324.8972569404635351 ) ) ;
#6751=CARTESIAN_POINT ( 'NONE',  ( 15.57127168073785128, 185.9592917570443262, 305.9563173247644272 ) ) ;
#6760=AXIS2_PLACEMENT_3D ( 'NONE', #8324, #15364, #10285 ) ;
#6785=CARTESIAN_POINT ( 'NONE',  ( 4.188990710115612970, 166.7868399227302518, 324.0943093659811325 ) ) ;
#6795=ADVANCED_FACE ( 'NONE', ( #11827 ), #4905, .F. ) ;
#6825=SURFACE_STYLE_FILL_AREA ( #14204 ) ;
#6827=CARTESIAN_POINT ( 'NONE',  ( 11.96119988344894658, 187.7040126267789049, 304.8853073998464538 ) ) ;
#6838=EDGE_CURVE ( 'NONE', #13470, #1967, #17692, .T. ) ;
#6841=CARTESIAN_POINT ( 'NONE',  ( 0.1821772113303683771, 327.3375983465229524, 315.3801061165882516 ) ) ;
#6857=CARTESIAN_POINT ( 'NONE',  ( 17.34172197772754132, 185.0087168425970106, 321.6195380205137440 ) ) ;
#6873=DIRECTION ( 'NONE',  ( -0.01292394549866727679, -0.005513023399720742325, -0.9999012842304692006 ) ) ;
#6887=CARTESIAN_POINT ( 'NONE',  ( 20.78937598082199756, 168.6311526966014185, 310.6889741221851295 ) ) ;
#6899=CARTESIAN_POINT ( 'NONE',  ( -8.330024601187750122, 185.3742117612894447, 323.2535488253523681 ) ) ;
#6910=CARTESIAN_POINT ( 'NONE',  ( 24.53513420042494886, 169.1064450938641244, 322.3183935679231240 ) ) ;
#6912=CARTESIAN_POINT ( 'NONE',  ( -28.23059182152518787, 324.0912873339099178, 316.1123282797007050 ) ) ;
#6920=ORIENTED_EDGE ( 'NONE', *, *, #19587, .F. ) ;
#6929=EDGE_CURVE ( 'NONE', #6678, #15431, #15598, .T. ) ;
#6933=CARTESIAN_POINT ( 'NONE',  ( 12.85290515736519090, 190.4809086768308362, 307.8507757859636627 ) ) ;
#6940=CARTESIAN_POINT ( 'NONE',  ( -9.891059059079783111, 187.9599303772540964, 308.1469373984825211 ) ) ;
#6976=CARTESIAN_POINT ( 'NONE',  ( 18.78219705323197886, 183.8529737559827311, 320.0839512733973038 ) ) ;
#6984=DIRECTION ( 'NONE',  ( 0.9934404589540162256, 0.1135548637187060589, -0.01346653032743021922 ) ) ;
#6988=EDGE_CURVE ( 'NONE', #126, #20005, #7402, .T. ) ;
#7003=CARTESIAN_POINT ( 'NONE',  ( -13.92525281995234820, 325.7770340667113942, 328.4523304068723064 ) ) ;
#7008=ORIENTED_EDGE ( 'NONE', *, *, #220, .T. ) ;
#7009=CARTESIAN_POINT ( 'NONE',  ( 20.88447817041588195, 168.6717208494654017, 318.0468511356601766 ) ) ;
#7033=CARTESIAN_POINT ( 'NONE',  ( -9.855893760047319319, 165.1672551789314127, 320.7685678595336185 ) ) ;
#7036=CARTESIAN_POINT ( 'NONE',  ( -10.92725181965738024, 335.2393912496561938, 320.3606194292975147 ) ) ;
#7041=ORIENTED_EDGE ( 'NONE', *, *, #14627, .F. ) ;
#7046=CARTESIAN_POINT ( 'NONE',  ( 16.51658783711441814, 187.6325752588389832, 308.9821593705616465 ) ) ;
#7058=CARTESIAN_POINT ( 'NONE',  ( 19.12444408178815891, 184.6244491382951480, 311.5251542095542732 ) ) ;
#7080=CARTESIAN_POINT ( 'NONE',  ( 12.27551321668195428, 188.3303010113484675, 320.9534237498031644 ) ) ;
#7091=CARTESIAN_POINT ( 'NONE',  ( -5.774671379064696630, 326.6239185723279661, 307.3367782756131419 ) ) ;
#7093=CARTESIAN_POINT ( 'NONE',  ( -14.87966828496393035, 178.9354977172588690, 312.8502022180878726 ) ) ;
#7096=CARTESIAN_POINT ( 'NONE',  ( 19.30212114139425594, 183.2083992702308137, 309.5025285114336384 ) ) ;
#7128=CARTESIAN_POINT ( 'NONE',  ( -0.7507300172562465512, 327.2392735797590717, 317.4522180588296578 ) ) ;
#7136=VERTEX_POINT ( 'NONE', #19663 ) ;
#7151=CARTESIAN_POINT ( 'NONE',  ( -13.50807349407477886, 164.7335820102402693, 316.8006659633929303 ) ) ;
#7163=CARTESIAN_POINT ( 'NONE',  ( 14.29282774033867831, 189.5286527345450338, 308.0677346475730474 ) ) ;
#7164=EDGE_CURVE ( 'NONE', #17417, #3170, #7764, .T. ) ;
#7173=CARTESIAN_POINT ( 'NONE',  ( 13.02821242091870424, 190.3077089839192695, 320.8514904664418737 ) ) ;
#7176=CARTESIAN_POINT ( 'NONE',  ( 18.21242699821856448, 184.1333206525301875, 308.0386800383396917 ) ) ;
#7206=CARTESIAN_POINT ( 'NONE',  ( -5.194761585865951936, 326.6903935298140027, 307.3756461515444585 ) ) ;
#7207=CARTESIAN_POINT ( 'NONE',  ( -14.85968324574364452, 178.8445255148678541, 318.6896797951268923 ) ) ;
#7210=CARTESIAN_POINT ( 'NONE',  ( 20.16435332678968706, 182.3960463823266878, 311.2982132828925614 ) ) ;
#7211=ORIENTED_EDGE ( 'NONE', *, *, #3608, .F. ) ;
#7217=DIRECTION ( 'NONE',  ( 0.9506032891036972909, -0.3102281881984320644, -0.01057629388542894074 ) ) ;
#7233=CARTESIAN_POINT ( 'NONE',  ( 21.53177455942607921, 168.7406653857994456, 316.7880417924246785 ) ) ;
#7251=VECTOR ( 'NONE', #17577, 1000.000000000000227 ) ;
#7254=CARTESIAN_POINT ( 'NONE',  ( -27.37946785251584103, 324.1954850279340121, 317.8131825257059973 ) ) ;
#7265=CARTESIAN_POINT ( 'NONE',  ( 18.87286229185910358, 185.1068706869312734, 317.5975223423299099 ) ) ;
#7276=SURFACE_STYLE_USAGE ( .BOTH. , #20947 ) ;
#7278=CARTESIAN_POINT ( 'NONE',  ( 17.77085107348584714, 184.5354884815143635, 309.5757466669096516 ) ) ;
#7283=CARTESIAN_POINT ( 'NONE',  ( -9.234393433859628075, 186.8255024611774502, 321.3851115294108354 ) ) ;
#7305=CARTESIAN_POINT ( 'NONE',  ( -9.998272952413007175, 187.5299746390215603, 321.1462410811432164 ) ) ;
#7311=CARTESIAN_POINT ( 'NONE',  ( -15.18074383830488294, 179.4905375618960477, 314.9769008739356764 ) ) ;
#7313=CARTESIAN_POINT ( 'NONE',  ( -2.669360985930898433, 326.9830943121846190, 308.3414884390720090 ) ) ;
#7314=CARTESIAN_POINT ( 'NONE',  ( -14.41394558013555560, 181.3065684521603202, 318.0453326090317319 ) ) ;
#7319=CARTESIAN_POINT ( 'NONE',  ( 11.85578982808163495, 187.7458312107169434, 305.0703088229346918 ) ) ;
#7330=ORIENTED_EDGE ( 'NONE', *, *, #125, .F. ) ;
#7342=CARTESIAN_POINT ( 'NONE',  ( 20.04619608162330024, 168.5799960362341210, 319.0729041454727621 ) ) ;
#7365=CARTESIAN_POINT ( 'NONE',  ( -12.91084759039031127, 164.8071687891488750, 318.1111553772653338 ) ) ;
#7373=CIRCLE ( 'NONE', #20199, 1.999999999999998224 ) ;
#7380=CARTESIAN_POINT ( 'NONE',  ( 17.75217047904729384, 186.5091196593482721, 318.8417065694452504 ) ) ;
#7395=CARTESIAN_POINT ( 'NONE',  ( 19.46619799173079812, 184.1572589165842260, 312.1803994612432120 ) ) ;
#7402=CIRCLE ( 'NONE', #16602, 10.71774939102741264 ) ;
#7429=CARTESIAN_POINT ( 'NONE',  ( -9.904114228265054720, 184.8598382391072619, 321.2234604397826843 ) ) ;
#7437=CARTESIAN_POINT ( 'NONE',  ( -14.91916526940173782, 178.8222960241703845, 316.3378698738634398 ) ) ;
#7444=CARTESIAN_POINT ( 'NONE',  ( 11.87689086465382715, 187.8426365274682439, 305.6410650122883794 ) ) ;
#7507=CARTESIAN_POINT ( 'NONE',  ( 19.94236535209076422, 183.5044621163393685, 314.4921078799457064 ) ) ;
#7516=CARTESIAN_POINT ( 'NONE',  ( -22.49358496127553053, 324.7653478115767030, 320.5678661935268678 ) ) ;
#7518=CARTESIAN_POINT ( 'NONE',  ( 19.63801391595304935, 182.9631121645107044, 312.1752918911519714 ) ) ;
#7526=CARTESIAN_POINT ( 'NONE',  ( -9.804288294571927409, 187.7022783261437837, 321.1616740932373091 ) ) ;
#7534=EDGE_CURVE ( 'NONE', #1183, #13714, #3002, .T. ) ;
#7540=CARTESIAN_POINT ( 'NONE',  ( -9.829296516163982034, 187.6860858752735908, 321.1599732488574546 ) ) ;
#7548=CARTESIAN_POINT ( 'NONE',  ( -9.773826842965361195, 187.7219482422972590, 321.1637457204829502 ) ) ;
#7552=CARTESIAN_POINT ( 'NONE',  ( -14.41756379550612799, 181.3026149279955632, 318.0496679571880918 ) ) ;
#7555=CARTESIAN_POINT ( 'NONE',  ( -15.14343016516442120, 179.5770291343474696, 315.4979406396071226 ) ) ;
#7573=CARTESIAN_POINT ( 'NONE',  ( 12.91228556302839792, 190.0204481364067988, 320.8669068103490076 ) ) ;
#7586=ORIENTED_EDGE ( 'NONE', *, *, #6929, .F. ) ;
#7588=CARTESIAN_POINT ( 'NONE',  ( -8.562029719258356764, 342.2165115496170529, 328.2923693891043513 ) ) ;
#7619=CARTESIAN_POINT ( 'NONE',  ( 19.60796286561798496, 183.9592037085494383, 312.5281987576885854 ) ) ;
#7636=LINE ( 'NONE', #2598, #20650 ) ;
#7642=CARTESIAN_POINT ( 'NONE',  ( -9.736871716074000815, 187.7457344247829667, 321.1662588281238868 ) ) ;
#7652=CARTESIAN_POINT ( 'NONE',  ( -10.92760325396984022, 186.9328588273032210, 308.3314949570851127 ) ) ;
#7658=CARTESIAN_POINT ( 'NONE',  ( 12.03061627106288967, 188.3248577112672706, 306.6667676847338271 ) ) ;
#7697=CARTESIAN_POINT ( 'NONE',  ( 4.150218873619613724, 166.7703008525310793, 321.0946055132897072 ) ) ;
#7706=CARTESIAN_POINT ( 'NONE',  ( 26.52201511833298397, 169.3335548213015329, 322.2914605072682548 ) ) ;
#7715=VERTEX_POINT ( 'NONE', #13018 ) ;
#7718=AXIS2_PLACEMENT_3D ( 'NONE', #13664, #22340, #6638 ) ;
#7731=EDGE_CURVE ( 'NONE', #9852, #9497, #17723, .T. ) ;
#7741=CARTESIAN_POINT ( 'NONE',  ( 20.32472999537270653, 182.3369386323682875, 317.0014608700818144 ) ) ;
#7764=CIRCLE ( 'NONE', #6660, 10.99999999999999822 ) ;
#7778=CARTESIAN_POINT ( 'NONE',  ( -14.46581794479437910, 179.5756009467052365, 311.6243789545613367 ) ) ;
#7789=AXIS2_PLACEMENT_3D ( 'NONE', #538, #6361, #19685 ) ;
#7796=CARTESIAN_POINT ( 'NONE',  ( -13.25750401672744161, 181.1680438727101432, 307.7338533305215833 ) ) ;
#7797=AXIS2_PLACEMENT_3D ( 'NONE', #9538, #22147, #939 ) ;
#7809=CARTESIAN_POINT ( 'NONE',  ( -8.671153205961791954, 185.7650231504708529, 306.6267288985166601 ) ) ;
#7816=ORIENTED_EDGE ( 'NONE', *, *, #12891, .F. ) ;
#7836=ORIENTED_EDGE ( 'NONE', *, *, #3343, .F. ) ;
#7850=CARTESIAN_POINT ( 'NONE',  ( 13.76389349044818644, 189.8999012668466833, 307.9600247906288928 ) ) ;
#7859=CARTESIAN_POINT ( 'NONE',  ( 20.69885819030740493, 181.8884547447338207, 314.5091122468493268 ) ) ;
#7868=AXIS2_PLACEMENT_3D ( 'NONE', #3633, #17556, #13769 ) ;
#7886=CARTESIAN_POINT ( 'NONE',  ( -8.381044803055207382, 185.3405392432284202, 323.2524327434741167 ) ) ;
#7892=CARTESIAN_POINT ( 'NONE',  ( -11.36165660420419066, 186.4279686652184012, 308.4742914312953985 ) ) ;
#7898=CARTESIAN_POINT ( 'NONE',  ( 12.74721152739840058, 190.3162922845854439, 307.8428787392024333 ) ) ;
#7899=ORIENTED_EDGE ( 'NONE', *, *, #18070, .F. ) ;
#7904=CARTESIAN_POINT ( 'NONE',  ( 12.69681717808449406, 190.5419464543700485, 307.8407304119797345 ) ) ;
#7905=CARTESIAN_POINT ( 'NONE',  ( -12.01575389183062192, 182.4076787623453129, 322.7174846376778987 ) ) ;
#7926=CARTESIAN_POINT ( 'NONE',  ( 13.43154693195699068, 190.0791210297336988, 320.8088049362866059 ) ) ;
#7944=CARTESIAN_POINT ( 'NONE',  ( 12.84373220155140949, 190.4863343871390953, 307.8501923929725876 ) ) ;
#7960=CARTESIAN_POINT ( 'NONE',  ( 19.94248262068743571, 183.5029939364791858, 314.4424437290580840 ) ) ;
#7973=ORIENTED_EDGE ( 'NONE', *, *, #11972, .F. ) ;
#7975=DIRECTION ( 'NONE',  ( 0.9934404589540162256, 0.1135548637187060589, -0.01346653032743021922 ) ) ;
#7995=CARTESIAN_POINT ( 'NONE',  ( -13.21851778092264240, 183.7781430057642922, 309.6523260561946245 ) ) ;
#8033=LINE ( 'NONE', #15067, #18412 ) ;
#8059=AXIS2_PLACEMENT_3D ( 'NONE', #9911, #3468, #17494 ) ;
#8075=CARTESIAN_POINT ( 'NONE',  ( 17.56092566177725800, 186.7283010723397751, 319.0062387086613285 ) ) ;
#8077=DIRECTION ( 'NONE',  ( -0.01292394549866742078, -0.005513023399720777019, -0.9999012842304693116 ) ) ;
#8094=CIRCLE ( 'NONE', #20920, 8.520833333333289517 ) ;
#8120=CARTESIAN_POINT ( 'NONE',  ( -13.32411518825262853, 183.5971624586300948, 309.7568532065889713 ) ) ;
#8155=VERTEX_POINT ( 'NONE', #6177 ) ;
#8171=CARTESIAN_POINT ( 'NONE',  ( -4.720905924553975730, 165.6695212782702811, 299.7132133896669188 ) ) ;
#8203=CARTESIAN_POINT ( 'NONE',  ( 15.62064282387073710, 186.1419012809306253, 320.4776025279708733 ) ) ;
#8214=ORIENTED_EDGE ( 'NONE', *, *, #14431, .T. ) ;
#8244=( BOUNDED_SURFACE ( )  B_SPLINE_SURFACE ( 3, 2, ( 
 ( #5111, #2952, #17439 ),
 ( #4771, #10422, #8670 ),
 ( #22226, #6518, #17196 ),
 ( #8450, #10090, #10194 ),
 ( #12031, #6629, #17102 ),
 ( #20748, #10307, #1364 ),
 ( #8340, #13652, #1472 ),
 ( #22449, #6741, #13765 ),
 ( #5002, #19018, #3280 ),
 ( #20970, #12723, #5228 ),
 ( #1921, #12382, #19363 ),
 ( #5689, #5454, #10531 ),
 ( #19689, #17672, #12268 ),
 ( #13982, #16184, #15719 ),
 ( #8908, #7080, #3958 ),
 ( #12610, #2133, #19255 ),
 ( #10981, #2031, #21090 ),
 ( #9132, #5579, #15957 ) ),
 .UNSPECIFIED., .F., .F., .T. ) 
 B_SPLINE_SURFACE_WITH_KNOTS ( ( 4, 2, 2, 2, 2, 2, 2, 2, 4 ),
 ( 3, 3 ),
 ( 0.08392082777195179755, 0.08669808355441036007, 0.08808671144563964828, 0.08878102539125429238, 0.08912818236406161443, 0.08930176085046526158, 0.08934515547206617336, 0.08938855009366708515, 0.08947533933686892260 ),
 ( 0.000000000000000000, 1.000000000000000000 ),
 .UNSPECIFIED. ) 
 GEOMETRIC_REPRESENTATION_ITEM ( )  RATIONAL_B_SPLINE_SURFACE ( (
 ( 1.000000000000000000, 0.8227386401547606143, 1.000000000000000000),
 ( 1.000000000000000000, 0.8263415838640109090, 1.000000000000000000),
 ( 1.000000000000000000, 0.8288608359785593072, 1.000000000000000000),
 ( 1.000000000000000000, 0.8282189721136420379, 1.000000000000000000),
 ( 1.000000000000000000, 0.8271574078587653478, 1.000000000000000000),
 ( 1.000000000000000000, 0.8239197622725578096, 1.000000000000000000),
 ( 1.000000000000000000, 0.8225730560359920673, 1.000000000000000000),
 ( 1.000000000000000000, 0.8201245374487728945, 1.000000000000000000),
 ( 1.000000000000000000, 0.8192370252838325762, 1.000000000000000000),
 ( 1.000000000000000000, 0.8177961922896359592, 1.000000000000000000),
 ( 1.000000000000000000, 0.8172976608657051001, 1.000000000000000000),
 ( 1.000000000000000000, 0.8166514735311385387, 1.000000000000000000),
 ( 1.000000000000000000, 0.8167936669053370569, 1.000000000000000000),
 ( 1.000000000000000000, 0.8168953424619973536, 1.000000000000000000),
 ( 1.000000000000000000, 0.8169461963296643647, 1.000000000000000000),
 ( 1.000000000000000000, 0.8170988061662717294, 1.000000000000000000),
 ( 1.000000000000000000, 0.8172006103767126550, 1.000000000000000000),
 ( 1.000000000000000000, 0.8173024788409366526, 1.000000000000000000) ) ) 
 REPRESENTATION_ITEM ( '' )  SURFACE ( )  );
#8246=CARTESIAN_POINT ( 'NONE',  ( -2.679299502224010254, 326.9817443121281713, 308.2885977099632555 ) ) ;
#8259=B_SPLINE_CURVE_WITH_KNOTS ( 'NONE', 3,
 ( #9468, #11213, #20132, #4405 ),
 .UNSPECIFIED., .F., .F.,
 ( 4, 4 ),
 ( 0.000000000000000000, 0.0001170083130068365703 ),
 .UNSPECIFIED. ) ;
#8261=CARTESIAN_POINT ( 'NONE',  ( -24.08933336292039229, 324.5818098845193731, 320.3078767544336642 ) ) ;
#8283=CARTESIAN_POINT ( 'NONE',  ( 12.82628922073134170, 190.6145596806321407, 307.8497150165550238 ) ) ;
#8299=EDGE_CURVE ( 'NONE', #6442, #5484, #17266, .T. ) ;
#8305=CARTESIAN_POINT ( 'NONE',  ( 12.16442896649338223, 187.7168230983759543, 322.9757373289252200 ) ) ;
#8324=CARTESIAN_POINT ( 'NONE',  ( 4.177359159166812219, 166.7818782016704802, 323.1943982101736879 ) ) ;
#8329=CARTESIAN_POINT ( 'NONE',  ( -8.301606475021044318, 185.5510420931183546, 308.0304484427728084 ) ) ;
#8340=CARTESIAN_POINT ( 'NONE',  ( 12.90979805384899848, 187.4290109168892968, 322.9333241855586607 ) ) ;
#8348=DIRECTION ( 'NONE',  ( -0.1136178953597578312, 0.9935164314186356593, -0.004009283626633664867 ) ) ;
#8352=CARTESIAN_POINT ( 'NONE',  ( -27.75997226120959382, 324.1497707426385659, 317.2680019637485316 ) ) ;
#8353=EDGE_CURVE ( 'NONE', #13470, #17822, #4385, .T. ) ;
#8358=EDGE_CURVE ( 'NONE', #18942, #17822, #21986, .T. ) ;
#8362=DIRECTION ( 'NONE',  ( 0.01292394549866727679, 0.005513023399720742325, 0.9999012842304692006 ) ) ;
#8365=CYLINDRICAL_SURFACE ( 'NONE', #18059, 22.50000000000000000 ) ;
#8373=ADVANCED_FACE ( 'NONE', ( #1480 ), #4907, .T. ) ;
#8390=EDGE_CURVE ( 'NONE', #13470, #5262, #22457, .T. ) ;
#8395=AXIS2_PLACEMENT_3D ( 'NONE', #21428, #17899, #16066 ) ;
#8426=CARTESIAN_POINT ( 'NONE',  ( 13.01890817498768449, 190.3110758050131892, 320.8522954438618058 ) ) ;
#8439=CARTESIAN_POINT ( 'NONE',  ( -9.804288294571927409, 187.7022783261437837, 321.1616740932373091 ) ) ;
#8446=CARTESIAN_POINT ( 'NONE',  ( -0.9086064320094255908, 327.1909312704538024, 309.9468142364838741 ) ) ;
#8450=CARTESIAN_POINT ( 'NONE',  ( 14.04062050856939337, 186.9464262198503377, 322.8169914968837588 ) ) ;
#8458=CARTESIAN_POINT ( 'NONE',  ( 3.982207582136937596, 166.6986315483347028, 308.0958888182936448 ) ) ;
#8475=AXIS2_PLACEMENT_3D ( 'NONE', #4245, #596, #9311 ) ;
#8507=EDGE_LOOP ( 'NONE', ( #18198, #5678, #12676, #4325, #20777, #11352, #8848, #1845 ) ) ;
#8508=DIRECTION ( 'NONE',  ( 0.3101392564284310427, 0.9506461370142480494, -0.009250070373107139796 ) ) ;
#8533=EDGE_CURVE ( 'NONE', #4095, #5262, #17247, .T. ) ;
#8546=CARTESIAN_POINT ( 'NONE',  ( 11.84242116924777299, 187.7489332779533981, 304.8764670816960347 ) ) ;
#8553=CARTESIAN_POINT ( 'NONE',  ( -8.612176237581371296, 185.3530072361552641, 305.1640391583723044 ) ) ;
#8563=PRODUCT_DEFINITION_CONTEXT ( 'detailed design', #12488, 'design' ) ;
#8583=CARTESIAN_POINT ( 'NONE',  ( 16.79209292077435123, 185.4001249148296893, 322.0628622613651260 ) ) ;
#8584=LINE ( 'NONE', #3426, #1651 ) ;
#8608=CARTESIAN_POINT ( 'NONE',  ( -5.563703806604336499, 326.7005119474492290, 320.3383740725300299 ) ) ;
#8610=CARTESIAN_POINT ( 'NONE',  ( -1.589012106048833584, 327.1475487665277342, 318.4782710686421865 ) ) ;
#8615=CARTESIAN_POINT ( 'NONE',  ( 3.872354045398264777, 166.6517708494370709, 299.5967279023346350 ) ) ;
#8634=CARTESIAN_POINT ( 'NONE',  ( -13.92525281995234820, 325.7770340667113942, 328.4523304068723064 ) ) ;
#8640=ORIENTED_EDGE ( 'NONE', *, *, #14627, .T. ) ;
#8652=CARTESIAN_POINT ( 'NONE',  ( 11.68933415262360676, 187.8362014856246560, 307.7594460564280894 ) ) ;
#8658=CARTESIAN_POINT ( 'NONE',  ( -8.403644388133985288, 185.4916053321884704, 305.1405741905838340 ) ) ;
#8667=CARTESIAN_POINT ( 'NONE',  ( -9.829296516163982034, 187.6860858752735908, 321.1599732488574546 ) ) ;
#8670=CARTESIAN_POINT ( 'NONE',  ( 15.88786633120246172, 188.4315875916928746, 320.0875345304690427 ) ) ;
#8683=CARTESIAN_POINT ( 'NONE',  ( 15.14609095036742481, 186.2064079090589814, 305.7394825653286148 ) ) ;
#8711=CARTESIAN_POINT ( 'NONE',  ( -2.528315839145332866, 327.0432605512580722, 319.2538853862658925 ) ) ;
#8717=DIRECTION ( 'NONE',  ( 0.9934404589540162256, 0.1135548637187057258, -0.01346653032742958084 ) ) ;
#8721=FACE_OUTER_BOUND ( 'NONE', #20341, .T. ) ;
#8732=CARTESIAN_POINT ( 'NONE',  ( -26.51496018000491617, 324.2983970019843696, 318.8161534577199632 ) ) ;
#8739=VERTEX_POINT ( 'NONE', #2730 ) ;
#8744=CARTESIAN_POINT ( 'NONE',  ( 19.75068821775290218, 183.8270873257126539, 315.7595470900485566 ) ) ;
#8757=CARTESIAN_POINT ( 'NONE',  ( 15.72063276321387093, 185.9256727956241377, 308.2960514488045192 ) ) ;
#8787=EDGE_CURVE ( 'NONE', #3170, #18739, #2606, .T. ) ;
#8790=CARTESIAN_POINT ( 'NONE',  ( -10.77448130880426724, 186.7844715323957416, 321.0194338377268650 ) ) ;
#8796=ORIENTED_EDGE ( 'NONE', *, *, #8787, .F. ) ;
#8800=CARTESIAN_POINT ( 'NONE',  ( -15.55825634263874413, 177.7403479327107618, 314.6945671552619501 ) ) ;
#8804=CARTESIAN_POINT ( 'NONE',  ( 17.16132609305713430, 185.1401191634033694, 321.7723388245965452 ) ) ;
#8830=FACE_OUTER_BOUND ( 'NONE', #6435, .T. ) ;
#8838=CARTESIAN_POINT ( 'NONE',  ( -5.692304260892842471, 326.6858542223808968, 320.3505014899224648 ) ) ;
#8848=ORIENTED_EDGE ( 'NONE', *, *, #20873, .T. ) ;
#8854=EDGE_LOOP ( 'NONE', ( #4733, #21539, #4951, #667 ) ) ;
#8859=CARTESIAN_POINT ( 'NONE',  ( -13.82219771749447368, 164.6877133068229284, 314.3360916636659681 ) ) ;
#8867=AXIS2_PLACEMENT_3D ( 'NONE', #13229, #4470, #11500 ) ;
#8874=ORIENTED_EDGE ( 'NONE', *, *, #10689, .T. ) ;
#8880=CARTESIAN_POINT ( 'NONE',  ( -16.00780723723847032, 316.4649337400251738, 414.4175034352881539 ) ) ;
#8888=CARTESIAN_POINT ( 'NONE',  ( 12.35205150687213127, 187.5852105437413400, 307.7116188629170779 ) ) ;
#8893=EDGE_CURVE ( 'NONE', #17682, #21571, #8094, .T. ) ;
#8908=CARTESIAN_POINT ( 'NONE',  ( 12.22168221341685879, 187.6955267389516564, 322.9731535519586032 ) ) ;
#8914=CARTESIAN_POINT ( 'NONE',  ( -8.736239094475285683, 185.1016632737992040, 323.2420184559757672 ) ) ;
#8925=CARTESIAN_POINT ( 'NONE',  ( -14.61876137247786112, 180.8472868627314369, 317.6002088574783784 ) ) ;
#8929=CARTESIAN_POINT ( 'NONE',  ( 20.45030313596652860, 182.1143970192508164, 312.2990932916914630 ) ) ;
#8946=DIRECTION ( 'NONE',  ( 0.3101392564284308762, 0.9506461370142480494, -0.009250070373106863975 ) ) ;
#8955=CARTESIAN_POINT ( 'NONE',  ( -0.1034336282460315837, 327.3082181160931441, 316.1934087155942166 ) ) ;
#8976=CARTESIAN_POINT ( 'NONE',  ( -13.33655421047878953, 164.7550532780195454, 317.2606976044711473 ) ) ;
#8979=EDGE_CURVE ( 'NONE', #3953, #15318, #10861, .T. ) ;
#8990=CARTESIAN_POINT ( 'NONE',  ( 19.88292633637799156, 183.6120083857789780, 315.1481641239921032 ) ) ;
#9002=CARTESIAN_POINT ( 'NONE',  ( 12.53471727977827044, 187.5120739667221699, 307.7020987390404230 ) ) ;
#9006=DIRECTION ( 'NONE',  ( -0.9934404589540165587, -0.1135548637187045462, 0.01346653032743214476 ) ) ;
#9026=CARTESIAN_POINT ( 'NONE',  ( -14.73958462865978980, 180.7047163397708971, 312.0297913800017113 ) ) ;
#9029=CARTESIAN_POINT ( 'NONE',  ( -13.46575745744828367, 183.1864814975198215, 319.4298558866661324 ) ) ;
#9036=CARTESIAN_POINT ( 'NONE',  ( -17.11750112564732618, 315.9920795429054010, 328.5475409320285962 ) ) ;
#9080=CARTESIAN_POINT ( 'NONE',  ( -9.069298571189188252, 165.2074204917897475, 308.4306052290647813 ) ) ;
#9094=CARTESIAN_POINT ( 'NONE',  ( 18.45279573939507145, 185.6574623812839491, 318.1353495108407969 ) ) ;
#9107=CARTESIAN_POINT ( 'NONE',  ( 13.04687021101641342, 190.3009381008880609, 320.8498765639175190 ) ) ;
#9109=CARTESIAN_POINT ( 'NONE',  ( 14.60385163837487532, 186.5550067726685484, 307.9188285726191339 ) ) ;
#9116=CARTESIAN_POINT ( 'NONE',  ( -8.943793367660859417, 186.3714091404604858, 321.6764070892438099 ) ) ;
#9132=CARTESIAN_POINT ( 'NONE',  ( 12.13657183616750679, 187.7271216158292759, 322.9769951237993268 ) ) ;
#9139=CARTESIAN_POINT ( 'NONE',  ( -9.258875922456445196, 185.4416665633954153, 321.2584118180014912 ) ) ;
#9143=CARTESIAN_POINT ( 'NONE',  ( -13.95813346672372468, 182.2598320623498580, 318.8173946239458587 ) ) ;
#9148=CARTESIAN_POINT ( 'NONE',  ( -12.86560286818836474, 181.5419395642671248, 319.9155313192819108 ) ) ;
#9154=CARTESIAN_POINT ( 'NONE',  ( 12.20664162007220099, 188.8323198333426376, 307.2129386106284983 ) ) ;
#9200=CARTESIAN_POINT ( 'NONE',  ( -7.685154071873219195, 165.4174906297564007, 321.2619620810605738 ) ) ;
#9231=CARTESIAN_POINT ( 'NONE',  ( 17.55321521090719727, 184.6409100556667795, 307.3691051642267666 ) ) ;
#9268=ORIENTED_EDGE ( 'NONE', *, *, #19877, .T. ) ;
#9270=CARTESIAN_POINT ( 'NONE',  ( -15.48395931107686074, 177.8963445608573295, 313.2677653863855767 ) ) ;
#9311=DIRECTION ( 'NONE',  ( -0.9934404589540163366, -0.1135548637187061005, 0.01346653032743037014 ) ) ;
#9349=CARTESIAN_POINT ( 'NONE',  ( 19.68743419676729189, 183.9263611086432775, 315.9693692526456630 ) ) ;
#9368=DIRECTION ( 'NONE',  ( 0.3101392564284310982, 0.9506461370142479383, -0.009250070373107712254 ) ) ;
#9382=CARTESIAN_POINT ( 'NONE',  ( -15.13015584224213228, 179.6094257463666679, 315.6214976206437655 ) ) ;
#9384=CARTESIAN_POINT ( 'NONE',  ( -15.00888604204753385, 180.0069015676392326, 312.9893017111969584 ) ) ;
#9400=CARTESIAN_POINT ( 'NONE',  ( 13.01890817498768449, 190.3110758050131892, 320.8522954438618058 ) ) ;
#9413=ORIENTED_EDGE ( 'NONE', *, *, #8390, .F. ) ;
#9455=CARTESIAN_POINT ( 'NONE',  ( 20.66208571675547745, 181.9457687355336759, 315.3755798616213042 ) ) ;
#9468=CARTESIAN_POINT ( 'NONE',  ( -9.804288294571927409, 187.7022783261437837, 321.1616740932373091 ) ) ;
#9495=CARTESIAN_POINT ( 'NONE',  ( -12.14916032298575921, 182.4209000231529672, 306.6034495403590086 ) ) ;
#9497=VERTEX_POINT ( 'NONE', #2388 ) ;
#9515=CARTESIAN_POINT ( 'NONE',  ( -12.37189876511640918, 182.1695727904451587, 306.8303737958513580 ) ) ;
#9524=AXIS2_PLACEMENT_3D ( 'NONE', #19130, #3071, #4893 ) ;
#9525=CARTESIAN_POINT ( 'NONE',  ( -8.542205542555748821, 185.5086388639571169, 305.9178550086769519 ) ) ;
#9538=CARTESIAN_POINT ( 'NONE',  ( 3.982207582136937596, 166.6986315483347028, 308.0958888182936448 ) ) ;
#9540=VECTOR ( 'NONE', #19480, 1000.000000000000227 ) ;
#9569=VECTOR ( 'NONE', #2929, 1000.000000000000000 ) ;
#9571=DIRECTION ( 'NONE',  ( 0.1136178953597579422, -0.9935164314186355483, 0.004009283626633659663 ) ) ;
#9579=EDGE_CURVE ( 'NONE', #13714, #22032, #3104, .T. ) ;
#9584=CARTESIAN_POINT ( 'NONE',  ( 19.41373208432103681, 183.2702314132801007, 319.1152548829093689 ) ) ;
#9617=CARTESIAN_POINT ( 'NONE',  ( -8.663799671886042830, 185.9178481321715424, 321.2345653191283645 ) ) ;
#9624=CARTESIAN_POINT ( 'NONE',  ( -14.77708621466310035, 180.6116793951536579, 312.1350740694625756 ) ) ;
#9633=CARTESIAN_POINT ( 'NONE',  ( 12.68111155422823266, 190.1386086654728160, 307.8189900089453772 ) ) ;
#9643=CARTESIAN_POINT ( 'NONE',  ( -9.397814517978851256, 184.8013626690785429, 305.2958327382877997 ) ) ;
#9664=CARTESIAN_POINT ( 'NONE',  ( 13.08556214908078985, 190.2789432977352533, 320.8465702879597643 ) ) ;
#9706=CARTESIAN_POINT ( 'NONE',  ( 19.05256028926003964, 183.6015641263033444, 317.6936443219116768 ) ) ;
#9738=CARTESIAN_POINT ( 'NONE',  ( -8.424310978314924370, 185.3118195958672345, 323.2514892018872956 ) ) ;
#9744=CARTESIAN_POINT ( 'NONE',  ( -13.52657357758894996, 183.2391904061878165, 309.9735533623801871 ) ) ;
#9748=VECTOR ( 'NONE', #14155, 1000.000000000000227 ) ;
#9754=CARTESIAN_POINT ( 'NONE',  ( 11.80916335469752987, 187.7920945708437728, 307.7671702419516464 ) ) ;
#9759=DIRECTION ( 'NONE',  ( 0.01292394549866745720, 0.005513023399720816918, 0.9999012842304693116 ) ) ;
#9773=CARTESIAN_POINT ( 'NONE',  ( 13.31679592837081572, 190.1462100374990030, 320.8234512119713031 ) ) ;
#9810=CARTESIAN_POINT ( 'NONE',  ( 20.07011326767535309, 182.6117360806082104, 317.7501157953450956 ) ) ;
#9823=EDGE_CURVE ( 'NONE', #17067, #17518, #11186, .T. ) ;
#9841=CARTESIAN_POINT ( 'NONE',  ( -14.59198460393170294, 181.0549870649192030, 311.6709863310374544 ) ) ;
#9852=VERTEX_POINT ( 'NONE', #8283 ) ;
#9854=CARTESIAN_POINT ( 'NONE',  ( -15.48458306684558394, 177.8487764627609238, 315.9761681140001883 ) ) ;
#9866=CARTESIAN_POINT ( 'NONE',  ( -8.967929144405097475, 186.2768650721423569, 307.3739889994579357 ) ) ;
#9903=CARTESIAN_POINT ( 'NONE',  ( 12.78871265281718728, 167.7718460055969274, 324.4777745207641146 ) ) ;
#9905=ORIENTED_EDGE ( 'NONE', *, *, #16398, .F. ) ;
#9911=CARTESIAN_POINT ( 'NONE',  ( -12.81536461602102683, 326.2504838843369726, 414.3222871145668478 ) ) ;
#9973=EDGE_CURVE ( 'NONE', #5484, #15351, #17243, .T. ) ;
#9985=CARTESIAN_POINT ( 'NONE',  ( -28.52776333611105386, 324.0526502209150976, 314.9593530838130278 ) ) ;
#10001=DIRECTION ( 'NONE',  ( -0.9506032891036972909, 0.3102281881984321754, 0.01057629388542893900 ) ) ;
#10024=LINE ( 'NONE', #9903, #22492 ) ;
#10074=TOROIDAL_SURFACE ( 'NONE', #16344, 17.29295143883736330, 7.000000000000003553 ) ;
#10087=CARTESIAN_POINT ( 'NONE',  ( -0.4653277981563680443, 327.2444197121904494, 310.6395216073121333 ) ) ;
#10088=CARTESIAN_POINT ( 'NONE',  ( -9.829246957410544994, 187.6861180068510464, 321.1599766194978542 ) ) ;
#10090=CARTESIAN_POINT ( 'NONE',  ( 13.75908793881580294, 187.5646522750408565, 320.9026951369706921 ) ) ;
#10093=EDGE_LOOP ( 'NONE', ( #14817, #9905, #13688, #15298, #12285 ) ) ;
#10111=FACE_OUTER_BOUND ( 'NONE', #10476, .T. ) ;
#10133=AXIS2_PLACEMENT_3D ( 'NONE', #14805, #17823, #3778 ) ;
#10156=CARTESIAN_POINT ( 'NONE',  ( -10.09063251380018400, 187.4441295575114168, 321.1374866210967980 ) ) ;
#10178=CARTESIAN_POINT ( 'NONE',  ( -9.831917787258822372, 187.9991244538465480, 308.1409416784720179 ) ) ;
#10194=CARTESIAN_POINT ( 'NONE',  ( 14.46615021700412740, 189.4447416640960569, 320.6057474549900803 ) ) ;
#10195=ORIENTED_EDGE ( 'NONE', *, *, #8893, .T. ) ;
#10205=CARTESIAN_POINT ( 'NONE',  ( -13.04685404786910574, 183.9066745433380845, 319.8387711160580125 ) ) ;
#10223=CARTESIAN_POINT ( 'NONE',  ( 3.872354045398264777, 166.6517708494370709, 299.5967279023346350 ) ) ;
#10243=ADVANCED_FACE ( 'NONE', ( #17385 ), #3571, .T. ) ;
#10250=DIRECTION ( 'NONE',  ( 0.9934404589540164476, 0.1135548637187057258, -0.01346653032743022095 ) ) ;
#10263=DIRECTION ( 'NONE',  ( -0.9999164797902017066, 0.000000000000000000, 0.01292414190463972781 ) ) ;
#10264=CARTESIAN_POINT ( 'NONE',  ( -9.959129957705535219, 187.5668473393425302, 321.1510774957479839 ) ) ;
#10267=AXIS2_PLACEMENT_3D ( 'NONE', #15724, #20936, #20977 ) ;
#10271=EDGE_LOOP ( 'NONE', ( #12710, #1281, #9268, #13133, #14861 ) ) ;
#10285=DIRECTION ( 'NONE',  ( -0.9934404589540162256, -0.1135548637187071275, 0.01346653032743056616 ) ) ;
#10307=CARTESIAN_POINT ( 'NONE',  ( 13.00038704669623613, 187.9860038210169364, 320.9566775397975107 ) ) ;
#10314=CARTESIAN_POINT ( 'NONE',  ( 12.78872557676268507, 167.7718515186203092, 324.4787744220483887 ) ) ;
#10319=CIRCLE ( 'NONE', #3700, 10.29357798165139393 ) ;
#10322=CARTESIAN_POINT ( 'NONE',  ( 16.40873467035000033, 185.6567299720572635, 322.3321779654820602 ) ) ;
#10337=LINE ( 'NONE', #20660, #20295 ) ;
#10346=AXIS2_PLACEMENT_3D ( 'NONE', #15848, #13771, #1811 ) ;
#10358=CARTESIAN_POINT ( 'NONE',  ( -5.649437442796671149, 326.6907401307370264, 320.3464590174583577 ) ) ;
#10369=CARTESIAN_POINT ( 'NONE',  ( -12.01575389183062192, 182.4076787623453129, 322.7174846376778987 ) ) ;
#10399=FILL_AREA_STYLE_COLOUR ( '', #3998 ) ;
#10401=CARTESIAN_POINT ( 'NONE',  ( 11.98344425196071761, 187.6955325895518172, 304.8869668606459413 ) ) ;
#10408=CARTESIAN_POINT ( 'NONE',  ( -10.01298669457304769, 187.8806077181497471, 308.1592502570636043 ) ) ;
#10410=ORIENTED_EDGE ( 'NONE', *, *, #17667, .F. ) ;
#10411=CIRCLE ( 'NONE', #18475, 2.272904689641356502 ) ;
#10422=CARTESIAN_POINT ( 'NONE',  ( 15.14365798081738745, 186.6008537337700659, 320.6317565638801739 ) ) ;
#10431=EDGE_LOOP ( 'NONE', ( #7586, #12006, #21426, #15879, #16956 ) ) ;
#10438=CARTESIAN_POINT ( 'NONE',  ( 14.26037014339171272, 186.6883954841667332, 305.3605431179787502 ) ) ;
#10448=CARTESIAN_POINT ( 'NONE',  ( -10.57022244108635256, 335.9790600926598927, 330.7543525966221409 ) ) ;
#10467=CARTESIAN_POINT ( 'NONE',  ( 20.23006072118110055, 168.5643786070652652, 309.9923577776485217 ) ) ;
#10476=EDGE_LOOP ( 'NONE', ( #6204, #5874, #22317, #13064 ) ) ;
#10486=ORIENTED_EDGE ( 'NONE', *, *, #9579, .F. ) ;
#10491=CARTESIAN_POINT ( 'NONE',  ( -11.91376962586675070, 164.8889363646316610, 310.1175901861107036 ) ) ;
#10506=CARTESIAN_POINT ( 'NONE',  ( 18.55084795937754905, 185.3714166030938770, 310.7056270676168310 ) ) ;
#10515=CARTESIAN_POINT ( 'NONE',  ( 12.08126718300561109, 187.6900170120506459, 307.7358539476931583 ) ) ;
#10531=CARTESIAN_POINT ( 'NONE',  ( 13.04191424503058450, 190.3037527154888551, 320.8502931330203296 ) ) ;
#10537=CARTESIAN_POINT ( 'NONE',  ( -8.992099355616254286, 184.9255222043797176, 323.2302142135638974 ) ) ;
#10544=CARTESIAN_POINT ( 'NONE',  ( -14.68167319698930129, 180.7010392265696908, 317.4437403699121205 ) ) ;
#10555=CARTESIAN_POINT ( 'NONE',  ( 4.855148840260169685, 158.0578537176658926, 299.6314082057050427 ) ) ;
#10572=CARTESIAN_POINT ( 'NONE',  ( -4.433483160726415129, 326.8290646393697898, 320.1652560256880520 ) ) ;
#10587=ORIENTED_EDGE ( 'NONE', *, *, #13962, .T. ) ;
#10590=FACE_OUTER_BOUND ( 'NONE', #14025, .T. ) ;
#10603=CARTESIAN_POINT ( 'NONE',  ( 19.94311012550880946, 183.4975381809269095, 314.2664455249164348 ) ) ;
#10617=CARTESIAN_POINT ( 'NONE',  ( 14.01676522198601660, 186.8106453161406648, 305.2787119402084386 ) ) ;
#10620=STYLED_ITEM ( 'NONE', ( #3718 ), #17529 ) ;
#10631=DIRECTION ( 'NONE',  ( 0.3101392564284315978, 0.9506461370142478273, -0.009250070373107145000 ) ) ;
#10644=CARTESIAN_POINT ( 'NONE',  ( -8.753245784830484766, 185.8505709766340317, 321.2394042940741770 ) ) ;
#10650=CARTESIAN_POINT ( 'NONE',  ( -14.11939326714681364, 181.9331570759241856, 318.5758607607144199 ) ) ;
#10654=CARTESIAN_POINT ( 'NONE',  ( -15.54784124399456502, 177.7690436490937316, 314.1134455231556331 ) ) ;
#10658=CARTESIAN_POINT ( 'NONE',  ( 15.77808660118132700, 185.8345873904136170, 306.0719219466911909 ) ) ;
#10689=EDGE_CURVE ( 'NONE', #4095, #11132, #18919, .T. ) ;
#10698=DIRECTION ( 'NONE',  ( 0.9506032891036977350, -0.3102281881984299550, -0.01057629388543066158 ) ) ;
#10700=DIRECTION ( 'NONE',  ( -0.3102455404053335308, -0.9506564598521395348, 0.000000000000000000 ) ) ;
#10711=CARTESIAN_POINT ( 'NONE',  ( -22.45062868030126779, 324.7702718825011630, 320.5707452954474661 ) ) ;
#10726=CARTESIAN_POINT ( 'NONE',  ( 18.22858106979587234, 185.9398809517860514, 318.3817688168216478 ) ) ;
#10739=CARTESIAN_POINT ( 'NONE',  ( 13.04683326300609636, 190.3009515221012862, 320.8498797597175667 ) ) ;
#10741=CARTESIAN_POINT ( 'NONE',  ( 17.45373000089112381, 184.7724903878686291, 309.3158825916956971 ) ) ;
#10749=CARTESIAN_POINT ( 'NONE',  ( -14.02864438394164459, 325.7329298795127670, 320.4531201330283352 ) ) ;
#10755=EDGE_CURVE ( 'NONE', #22032, #20005, #20014, .T. ) ;
#10769=CARTESIAN_POINT ( 'NONE',  ( -11.74988407969402360, 185.7573108837101756, 320.6989643996056998 ) ) ;
#10774=CARTESIAN_POINT ( 'NONE',  ( -13.52516265657463812, 183.2462493215299162, 309.9645816984750013 ) ) ;
#10778=CARTESIAN_POINT ( 'NONE',  ( -15.16713580098303638, 179.5535043013633754, 314.1163235527705524 ) ) ;
#10782=CARTESIAN_POINT ( 'NONE',  ( 20.38555108690226447, 182.1783941675930691, 312.0429188998837162 ) ) ;
#10805=ORIENTED_EDGE ( 'NONE', *, *, #8893, .F. ) ;
#10806=ORIENTED_EDGE ( 'NONE', *, *, #14009, .F. ) ;
#10815=CARTESIAN_POINT ( 'NONE',  ( -5.606570624700499827, 326.6956260390930993, 320.3424165449941938 ) ) ;
#10828=EDGE_LOOP ( 'NONE', ( #5100, #8214, #17725, #10806 ) ) ;
#10836=CARTESIAN_POINT ( 'NONE',  ( -23.79181689863955285, 324.5651258154593961, 307.7422675453725560 ) ) ;
#10847=CARTESIAN_POINT ( 'NONE',  ( -13.89421726780587996, 325.7902730365928505, 330.8534925327304563 ) ) ;
#10858=CARTESIAN_POINT ( 'NONE',  ( 20.02494354238641705, 182.5313087350443482, 310.9605567950519003 ) ) ;
#10861=B_SPLINE_CURVE_WITH_KNOTS ( 'NONE', 3,
 ( #7526, #16052, #290, #7283, #17653, #1902, #9116, #63, #5561, #14324, #408, #12370, #19675, #21295 ),
 .UNSPECIFIED., .F., .F.,
 ( 4, 2, 2, 2, 2, 2, 4 ),
 ( 0.000000000000000000, 0.0009165371227192408397, 0.001374805684078860175, 0.001833074245438479294, 0.002291342806798098413, 0.002749611368157717749, 0.003666148490876996752 ),
 .UNSPECIFIED. ) ;
#10879=CARTESIAN_POINT ( 'NONE',  ( -9.987580305889029120, 184.1998911412988207, 323.1427045197882535 ) ) ;
#10885=DIRECTION ( 'NONE',  ( -0.1136178953597578312, 0.9935164314186356593, -0.004009283626633664867 ) ) ;
#10887=CARTESIAN_POINT ( 'NONE',  ( -14.85578608565897518, 180.2907807798002295, 316.9594776086723300 ) ) ;
#10893=CARTESIAN_POINT ( 'NONE',  ( 4.195452682864946325, 166.7895964344300808, 324.5942600080963985 ) ) ;
#10905=EDGE_LOOP ( 'NONE', ( #1943, #17430, #20509, #16984, #14329 ) ) ;
#10915=CARTESIAN_POINT ( 'NONE',  ( -8.517247419455044266, 185.4376447080673529, 305.5391571354516600 ) ) ;
#10938=CARTESIAN_POINT ( 'NONE',  ( -28.54471604494488446, 324.0454186304925202, 313.6477539799737428 ) ) ;
#10948=CARTESIAN_POINT ( 'NONE',  ( 16.96733342230854902, 187.3721694870787076, 319.4512518112545649 ) ) ;
#10952=CARTESIAN_POINT ( 'NONE',  ( -12.86548928906161571, 326.2291019854885121, 410.4442357137708086 ) ) ;
#10959=CARTESIAN_POINT ( 'NONE',  ( -10.01777582550143642, 187.9231991978160750, 308.1591746062594552 ) ) ;
#10961=CARTESIAN_POINT ( 'NONE',  ( 14.48605119362585292, 189.3857847177796145, 308.1185926126519234 ) ) ;
#10965=( LENGTH_UNIT ( ) NAMED_UNIT ( * ) SI_UNIT ( .MILLI., .METRE. ) );
#10981=CARTESIAN_POINT ( 'NONE',  ( 12.16090316381096592, 187.7181452293938264, 322.9758963384301751 ) ) ;
#10990=ORIENTED_EDGE ( 'NONE', *, *, #138, .F. ) ;
#10991=CARTESIAN_POINT ( 'NONE',  ( -14.55445127856342680, 180.9963701914269336, 317.7651582568626054 ) ) ;
#10993=CARTESIAN_POINT ( 'NONE',  ( -15.09948650839594109, 178.4733586872830529, 317.9816280114638971 ) ) ;
#11001=CARTESIAN_POINT ( 'NONE',  ( 12.36865781294890532, 189.2856407680814641, 307.5221633547453166 ) ) ;
#11052=CARTESIAN_POINT ( 'NONE',  ( -17.63692254078916832, 314.5473693806632127, 324.2384804942064989 ) ) ;
#11081=CARTESIAN_POINT ( 'NONE',  ( 19.82458506650596419, 183.6531909117268526, 313.2672148072155096 ) ) ;
#11103=CARTESIAN_POINT ( 'NONE',  ( -22.49358496127894824, 324.7653478115763050, 320.5678661935266973 ) ) ;
#11123=CARTESIAN_POINT ( 'NONE',  ( -10.01711797457082831, 184.3274371752771685, 305.4743107222549270 ) ) ;
#11132=VERTEX_POINT ( 'NONE', #973 ) ;
#11150=CIRCLE ( 'NONE', #5643, 10.00000000000001421 ) ;
#11151=CARTESIAN_POINT ( 'NONE',  ( 11.85964614693714836, 187.7423844643599296, 304.8777488482054423 ) ) ;
#11154=ORIENTED_EDGE ( 'NONE', *, *, #17341, .F. ) ;
#11186=CIRCLE ( 'NONE', #17068, 2.999999999999999556 ) ;
#11199=CARTESIAN_POINT ( 'NONE',  ( 20.63696371470829760, 181.9335396870980048, 313.3533115342202677 ) ) ;
#11213=CARTESIAN_POINT ( 'NONE',  ( -9.826031587490524188, 187.7354486172501709, 321.1602828553623681 ) ) ;
#11228=CARTESIAN_POINT ( 'NONE',  ( -8.630726460828782365, 185.9406206071954841, 321.2368171913553283 ) ) ;
#11236=CARTESIAN_POINT ( 'NONE',  ( -14.82189735930671759, 179.0281877771801931, 312.6327372929670219 ) ) ;
#11239=CARTESIAN_POINT ( 'NONE',  ( -14.19665567542432072, 325.6612605753163621, 307.4544034380322728 ) ) ;
#11241=CARTESIAN_POINT ( 'NONE',  ( 12.31224524591022274, 189.1288638982456973, 307.4294852416394974 ) ) ;
#11249=CARTESIAN_POINT ( 'NONE',  ( -15.48725902187971215, 177.8900859623065571, 313.3020055068878946 ) ) ;
#11253=CARTESIAN_POINT ( 'NONE',  ( 12.66771380998468821, 189.3290151587127355, 321.0882186569899659 ) ) ;
#11279=CARTESIAN_POINT ( 'NONE',  ( -7.853344289118919797, 165.3457450004224540, 308.2494022372945324 ) ) ;
#11287=VERTEX_POINT ( 'NONE', #18544 ) ;
#11304=CARTESIAN_POINT ( 'NONE',  ( 19.47897356911659728, 183.1989695422251145, 316.9366591568934837 ) ) ;
#11336=AXIS2_PLACEMENT_3D ( 'NONE', #20322, #8362, #22143 ) ;
#11340=CARTESIAN_POINT ( 'NONE',  ( -10.83602898747849075, 183.6695850371822019, 308.2317009130024985 ) ) ;
#11346=EDGE_CURVE ( 'NONE', #5334, #18942, #3072, .T. ) ;
#11347=VECTOR ( 'NONE', #16407, 1000.000000000000227 ) ;
#11352=ORIENTED_EDGE ( 'NONE', *, *, #15237, .T. ) ;
#11354=CARTESIAN_POINT ( 'NONE',  ( -15.42064199597873753, 178.0145423516129881, 312.7841245303434903 ) ) ;
#11377=PLANE ( 'NONE',  #19125 ) ;
#11418=CARTESIAN_POINT ( 'NONE',  ( 18.15385362334754404, 184.3839151010789408, 320.8406986940494789 ) ) ;
#11422=( NAMED_UNIT ( * ) PLANE_ANGLE_UNIT ( ) SI_UNIT ( $, .RADIAN. ) );
#11429=CARTESIAN_POINT ( 'NONE',  ( 13.04687021101641342, 190.3009381008880609, 320.8498765639175190 ) ) ;
#11438=CARTESIAN_POINT ( 'NONE',  ( 4.169604791867612015, 166.7785703876306513, 322.5944574396354483 ) ) ;
#11440=DIRECTION ( 'NONE',  ( 0.09199399308265900077, -0.9957502728239346901, 0.004301093787334665970 ) ) ;
#11449=CARTESIAN_POINT ( 'NONE',  ( -9.810751399401715034, 187.6981029871982400, 321.1612345458386812 ) ) ;
#11459=CARTESIAN_POINT ( 'NONE',  ( -14.65122776820497918, 179.2857995626968943, 310.0431837285613028 ) ) ;
#11473=CARTESIAN_POINT ( 'NONE',  ( 11.91668050545732882, 187.7209081685431613, 304.8819943630518878 ) ) ;
#11474=CARTESIAN_POINT ( 'NONE',  ( -14.77971672006231252, 178.9662530012681714, 318.9012573015519934 ) ) ;
#11490=CARTESIAN_POINT ( 'NONE',  ( -9.044567292803851188, 186.4032078415717422, 307.5010082646681440 ) ) ;
#11500=DIRECTION ( 'NONE',  ( 0.9934404589540163366, 0.1135548637187048376, -0.01346653032743036667 ) ) ;
#11511=CARTESIAN_POINT ( 'NONE',  ( -14.02864438394168722, 325.7329298795136197, 320.4531201330285626 ) ) ;
#11512=DIRECTION ( 'NONE',  ( 0.9934404589540163366, 0.1135548637187060866, -0.01346653032743036840 ) ) ;
#11540=CARTESIAN_POINT ( 'NONE',  ( 20.66604384607886402, 181.9072547581223205, 313.6374335290682893 ) ) ;
#11568=CARTESIAN_POINT ( 'NONE',  ( -8.676042597691862923, 185.9097051440071766, 321.2330616462555781 ) ) ;
#11574=CARTESIAN_POINT ( 'NONE',  ( -13.87886915313458580, 180.3914499437145764, 310.5935113253086683 ) ) ;
#11586=EDGE_LOOP ( 'NONE', ( #11635, #22125, #4276, #14670, #10410 ) ) ;
#11588=CARTESIAN_POINT ( 'NONE',  ( 11.82412558468182873, 187.7865448877315657, 307.7681344816915612 ) ) ;
#11592=DIRECTION ( 'NONE',  ( -0.01292394549866745720, -0.005513023399720816918, -0.9999012842304692006 ) ) ;
#11635=ORIENTED_EDGE ( 'NONE', *, *, #22511, .T. ) ;
#11655=LINE ( 'NONE', #16952, #4087 ) ;
#11682=CARTESIAN_POINT ( 'NONE',  ( -8.449107425469586374, 185.4541341740502958, 308.0383059716917273 ) ) ;
#11700=ORIENTED_EDGE ( 'NONE', *, *, #9823, .T. ) ;
#11704=CARTESIAN_POINT ( 'NONE',  ( -27.84085044979666179, 324.1152701834824938, 311.0106090768176159 ) ) ;
#11739=EDGE_LOOP ( 'NONE', ( #13663, #20229, #16813, #21782, #5954 ) ) ;
#11747=EDGE_CURVE ( 'NONE', #5484, #5811, #11150, .T. ) ;
#11818=CARTESIAN_POINT ( 'NONE',  ( 3.872354045398264777, 166.6517708494370709, 299.5967279023346350 ) ) ;
#11819=AXIS2_PLACEMENT_3D ( 'NONE', #6308, #9759, #16775 ) ;
#11827=FACE_OUTER_BOUND ( 'NONE', #10828, .T. ) ;
#11832=CARTESIAN_POINT ( 'NONE',  ( -22.49358496127553053, 324.7653478115767030, 320.5678661935268678 ) ) ;
#11836=TOROIDAL_SURFACE ( 'NONE', #7789, 20.50000000000000355, 2.000000000000000000 ) ;
#11896=ORIENTED_EDGE ( 'NONE', *, *, #5020, .T. ) ;
#11930=CARTESIAN_POINT ( 'NONE',  ( -0.8096692839990790036, 327.2331353181372720, 317.6013947485918720 ) ) ;
#11940=CARTESIAN_POINT ( 'NONE',  ( -12.63436650347019885, 181.7513824828561440, 322.1994800631134694 ) ) ;
#11968=ORIENTED_EDGE ( 'NONE', *, *, #14587, .T. ) ;
#11972=EDGE_CURVE ( 'NONE', #5229, #21242, #2556, .T. ) ;
#11979=CARTESIAN_POINT ( 'NONE',  ( -10.88352610546617250, 183.4880351429991379, 323.0108604666241376 ) ) ;
#11995=ADVANCED_FACE ( 'NONE', ( #1368 ), #10074, .F. ) ;
#12006=ORIENTED_EDGE ( 'NONE', *, *, #16172, .F. ) ;
#12015=DIRECTION ( 'NONE',  ( -0.01292394549866745720, -0.005513023399720816918, -0.9999012842304692006 ) ) ;
#12016=CARTESIAN_POINT ( 'NONE',  ( -8.508136329860027658, 185.4226668845482209, 305.1523461349310082 ) ) ;
#12031=CARTESIAN_POINT ( 'NONE',  ( 13.67035244215019851, 187.1120429933681351, 322.8635577162621644 ) ) ;
#12044=CARTESIAN_POINT ( 'NONE',  ( 19.55320478417725738, 183.1354159283349929, 318.8669710253166159 ) ) ;
#12047=CARTESIAN_POINT ( 'NONE',  ( -10.73300451425737734, 335.5619885905173305, 328.3571198817161303 ) ) ;
#12055=CARTESIAN_POINT ( 'NONE',  ( 3.898201936395599532, 166.6627968962365287, 301.5965304707955852 ) ) ;
#12069=DIRECTION ( 'NONE',  ( 0.000000000000000000, 0.000000000000000000, 1.000000000000000000 ) ) ;
#12074=CARTESIAN_POINT ( 'NONE',  ( -2.536883864190021320, 327.0424951675884131, 319.3070269798304253 ) ) ;
#12082=DIRECTION ( 'NONE',  ( 0.9934404589540163366, 0.1135548637187052401, -0.01346653032743036320 ) ) ;
#12090=CARTESIAN_POINT ( 'NONE',  ( -12.72332588857627300, 326.2897452428853740, 421.4431498403059777 ) ) ;
#12123=CARTESIAN_POINT ( 'NONE',  ( 11.95378257394767196, 187.7068342974569362, 304.8847554649954645 ) ) ;
#12145=EDGE_LOOP ( 'NONE', ( #14505, #20668, #16907, #9413, #20910, #4713, #16498, #21472 ) ) ;
#12146=CARTESIAN_POINT ( 'NONE',  ( -12.86548928906161571, 326.2291019854885121, 410.4442357137708086 ) ) ;
#12155=DIRECTION ( 'NONE',  ( -0.01292394549866727679, -0.005513023399720742325, -0.9999012842304692006 ) ) ;
#12159=DIRECTION ( 'NONE',  ( -0.9934404589540163366, -0.1135548637187057258, 0.01346653032743036146 ) ) ;
#12163=CARTESIAN_POINT ( 'NONE',  ( 12.85102440982953809, 187.3455989732921694, 304.9938768930631454 ) ) ;
#12177=DIRECTION ( 'NONE',  ( -0.3102455404053308108, -0.9506564598521405340, 0.000000000000000000 ) ) ;
#12191=DIRECTION ( 'NONE',  ( -0.01292394549866745720, -0.005513023399720816918, -0.9999012842304692006 ) ) ;
#12200=CARTESIAN_POINT ( 'NONE',  ( 21.95462417325102322, 168.7812190940428536, 314.8544026679174408 ) ) ;
#12207=PLANE ( 'NONE',  #22127 ) ;
#12223=CARTESIAN_POINT ( 'NONE',  ( -28.46703706805638134, 324.0603700370125466, 315.1514505861725866 ) ) ;
#12234=CARTESIAN_POINT ( 'NONE',  ( 19.15702598245626831, 184.5830064527947059, 311.5659919418918093 ) ) ;
#12244=CARTESIAN_POINT ( 'NONE',  ( 11.85672047603351054, 187.7744756917181803, 307.7628753140074309 ) ) ;
#12256=ADVANCED_FACE ( 'NONE', ( #6744 ), #13027, .T. ) ;
#12257=EDGE_CURVE ( 'NONE', #17518, #5334, #3087, .T. ) ;
#12268=CARTESIAN_POINT ( 'NONE',  ( 13.02613253520115499, 190.3084650069641839, 320.8516703567468085 ) ) ;
#12275=CARTESIAN_POINT ( 'NONE',  ( -9.663116041263174694, 184.4449190506678633, 323.1798533313222492 ) ) ;
#12280=DIRECTION ( 'NONE',  ( 0.9934404589540163366, 0.1135548637187061005, -0.01346653032743037014 ) ) ;
#12285=ORIENTED_EDGE ( 'NONE', *, *, #8979, .F. ) ;
#12288=CARTESIAN_POINT ( 'NONE',  ( 18.46966468191076416, 183.9248624754537502, 308.3369342292732540 ) ) ;
#12319=CARTESIAN_POINT ( 'NONE',  ( -0.5070102419236742763, 327.2655426976345439, 317.0551077940115192 ) ) ;
#12331=DIRECTION ( 'NONE',  ( -0.1136178953597579422, 0.9935164314186355483, -0.004009283626633659663 ) ) ;
#12339=CARTESIAN_POINT ( 'NONE',  ( -13.74451874060598122, 164.7026647133428980, 315.8397882698648687 ) ) ;
#12352=CARTESIAN_POINT ( 'NONE',  ( 16.68734734459444269, 187.6588240762195028, 319.6336511773113784 ) ) ;
#12364=CARTESIAN_POINT ( 'NONE',  ( 15.35300465305828510, 186.1419466745651334, 308.1514022875052774 ) ) ;
#12370=CARTESIAN_POINT ( 'NONE',  ( -8.447676300393007764, 185.5761720159400738, 322.6786239791117623 ) ) ;
#12382=CARTESIAN_POINT ( 'NONE',  ( 12.37582071282576024, 188.2881946015995709, 320.9507921273384454 ) ) ;
#12384=CARTESIAN_POINT ( 'NONE',  ( -22.49358496127894824, 324.7653478115763050, 320.5678661935266973 ) ) ;
#12397=CARTESIAN_POINT ( 'NONE',  ( -14.77271874809119900, 178.9768699339249451, 318.9195234373038375 ) ) ;
#12404=CARTESIAN_POINT ( 'NONE',  ( -10.89787692332478386, 335.2519218263954599, 322.6332997474033277 ) ) ;
#12440=CARTESIAN_POINT ( 'NONE',  ( -11.29548081222967326, 164.9574442151662197, 309.5726054092390314 ) ) ;
#12467=CARTESIAN_POINT ( 'NONE',  ( 12.66469053819756496, 187.4244128634429956, 304.9628814567714699 ) ) ;
#12473=CIRCLE ( 'NONE', #9524, 11.78759343285143224 ) ;
#12488=APPLICATION_CONTEXT ( 'automotive_design' ) ;
#12497=CARTESIAN_POINT ( 'NONE',  ( -11.49273635071671862, 182.9480784776224880, 322.8740417677803407 ) ) ;
#12502=CARTESIAN_POINT ( 'NONE',  ( -12.72040503869455286, 184.6056756926249989, 309.1932742806828287 ) ) ;
#12504=CARTESIAN_POINT ( 'NONE',  ( -3.646887971868283618, 326.8692299522281814, 307.8272933952192716 ) ) ;
#12505=CARTESIAN_POINT ( 'NONE',  ( -14.49142894009190741, 179.3925286715590346, 319.5713301818169043 ) ) ;
#12507=CARTESIAN_POINT ( 'NONE',  ( 19.43357779880557601, 183.2511996782348547, 319.0807864945002166 ) ) ;
#12532=CARTESIAN_POINT ( 'NONE',  ( 0.05613562462218960047, 327.3245918075140821, 315.7288890211281682 ) ) ;
#12538=B_SPLINE_SURFACE_WITH_KNOTS ( 'NONE', 3, 1, ( 
 ( #19650, #1865 ),
 ( #5299, #9200 ),
 ( #10711, #5645 ),
 ( #21373, #17502 ),
 ( #3817, #14410 ),
 ( #5181, #1754 ),
 ( #3580, #7033 ),
 ( #19319, #3917 ),
 ( #20927, #17859 ),
 ( #16024, #17615 ),
 ( #8732, #17743 ),
 ( #22616, #13933 ),
 ( #7254, #1988 ),
 ( #21256, #7365 ),
 ( #14061, #8976 ),
 ( #6912, #7151 ),
 ( #12223, #12339 ),
 ( #2197, #12680 ),
 ( #10938, #8859 ),
 ( #15908, #19207 ),
 ( #261, #17961 ),
 ( #152, #3690 ),
 ( #14178, #3477 ),
 ( #14283, #5524 ),
 ( #21155, #5403 ),
 ( #21046, #10491 ),
 ( #2095, #12440 ),
 ( #19429, #15786 ),
 ( #12555, #19549 ),
 ( #372, #26 ),
 ( #10836, #9080 ),
 ( #16131, #16704 ),
 ( #16468, #4142 ),
 ( #21585, #12779 ),
 ( #14523, #11279 ),
 ( #18402, #838 ) ),
 .UNSPECIFIED., .F., .F., .F.,
 ( 4, 3, 2, 2, 2, 2, 2, 2, 2, 2, 2, 2, 2, 2, 2, 3, 4 ),
 ( 2, 2 ),
 ( -0.01000000000000000021, 0.000000000000000000, 0.1250000000000000278, 0.1875000000000000555, 0.2500000000000000555, 0.3125000000000000555, 0.3750000000000001110, 0.4375000000000001110, 0.5000000000000001110, 0.5625000000000001110, 0.6250000000000001110, 0.6875000000000001110, 0.7500000000000002220, 0.8125000000000002220, 0.8750000000000002220, 1.000000000000000000, 1.010000000000000009 ),
 ( 0.000000000000000000, 1.000000000000000000 ),
 .UNSPECIFIED. ) ;
#12555=CARTESIAN_POINT ( 'NONE',  ( -25.05452705409702574, 324.4228452382362775, 308.2681417827414521 ) ) ;
#12572=TOROIDAL_SURFACE ( 'NONE', #18110, 20.50000000000000355, 2.000000000000000000 ) ;
#12586=CARTESIAN_POINT ( 'NONE',  ( 19.81846420101658879, 182.7288148374562411, 310.4831695857175760 ) ) ;
#12610=CARTESIAN_POINT ( 'NONE',  ( 12.18522217402714070, 187.7091244767421188, 322.9747985970192872 ) ) ;
#12611=ORIENTED_EDGE ( 'NONE', *, *, #13218, .F. ) ;
#12622=CARTESIAN_POINT ( 'NONE',  ( -15.07023257787665749, 179.7582508136519266, 316.0339885398511797 ) ) ;
#12628=CARTESIAN_POINT ( 'NONE',  ( 19.29271048405903244, 168.4538167080974063, 309.1579687774811305 ) ) ;
#12629=CARTESIAN_POINT ( 'NONE',  ( -15.49848325445370989, 177.8265085296330028, 315.8457734436829583 ) ) ;
#12668=CARTESIAN_POINT ( 'NONE',  ( -13.99926948760909795, 325.7454604562529425, 322.7258004511344325 ) ) ;
#12676=ORIENTED_EDGE ( 'NONE', *, *, #8358, .F. ) ;
#12680=CARTESIAN_POINT ( 'NONE',  ( -13.80923234909357333, 164.6932440001694431, 315.3391977597048594 ) ) ;
#12703=CARTESIAN_POINT ( 'NONE',  ( 16.78432341940586880, 185.2449657461795027, 308.8478038024924217 ) ) ;
#12710=ORIENTED_EDGE ( 'NONE', *, *, #9973, .F. ) ;
#12723=CARTESIAN_POINT ( 'NONE',  ( 12.41521462045219693, 188.2702244292405283, 320.9524563331297031 ) ) ;
#12734=CARTESIAN_POINT ( 'NONE',  ( -14.18436105576317985, 179.8295574832275463, 320.1833246747981434 ) ) ;
#12767=ORIENTED_EDGE ( 'NONE', *, *, #16295, .T. ) ;
#12779=CARTESIAN_POINT ( 'NONE',  ( -7.896211107215091118, 165.3408590920663244, 308.2534447097586963 ) ) ;
#12780=CARTESIAN_POINT ( 'NONE',  ( -10.02117361870881851, 187.8727420016839176, 308.1601407300097435 ) ) ;
#12806=CARTESIAN_POINT ( 'NONE',  ( 20.11979018982224687, 182.4391765495445838, 311.2061076290632968 ) ) ;
#12842=CARTESIAN_POINT ( 'NONE',  ( -14.34549876140896174, 179.6624466946600194, 317.9627730398437393 ) ) ;
#12865=CIRCLE ( 'NONE', #18715, 10.00000000000001421 ) ;
#12887=CARTESIAN_POINT ( 'NONE',  ( 4.195452682864946325, 166.7895964344300808, 324.5942600080963985 ) ) ;
#12891=EDGE_CURVE ( 'NONE', #21571, #8155, #16553, .T. ) ;
#12932=TOROIDAL_SURFACE ( 'NONE', #4094, 10.00000000000000178, 2.272904689641331188 ) ;
#12933=CARTESIAN_POINT ( 'NONE',  ( 18.80756281266039665, 183.8219316425800685, 318.0440155801259721 ) ) ;
#12939=APPLICATION_CONTEXT ( 'automotive_design' ) ;
#12942=CARTESIAN_POINT ( 'NONE',  ( -10.01265065029762980, 187.8784833776788332, 308.1592754748398875 ) ) ;
#12973=CARTESIAN_POINT ( 'NONE',  ( -9.373580856408977979, 184.8150131700745646, 307.9996070035269327 ) ) ;
#12990=CARTESIAN_POINT ( 'NONE',  ( -15.56353044989331735, 177.7370943402667649, 314.3607490585801543 ) ) ;
#12994=CARTESIAN_POINT ( 'NONE',  ( -19.28847592064633787, 309.3375565838056787, 328.6122914246403184 ) ) ;
#13017=DIRECTION ( 'NONE',  ( 0.9934404589540163366, 0.1135548637187057258, -0.01346653032743021922 ) ) ;
#13018=CARTESIAN_POINT ( 'NONE',  ( 11.48281922048859727, 176.2279375523750957, 299.4455621116320003 ) ) ;
#13027=TOROIDAL_SURFACE ( 'NONE', #7868, -102.0000000000000000, 120.0000000000000000 ) ;
#13055=CARTESIAN_POINT ( 'NONE',  ( 19.41230309865470716, 184.3421512348843692, 316.6627316332904343 ) ) ;
#13064=ORIENTED_EDGE ( 'NONE', *, *, #4686, .T. ) ;
#13068=CARTESIAN_POINT ( 'NONE',  ( 12.46561401535050528, 167.6340204206038891, 299.4802424150023512 ) ) ;
#13087=CARTESIAN_POINT ( 'NONE',  ( -14.08815279242220520, 180.1090064943867333, 310.9205019102012670 ) ) ;
#13101=CARTESIAN_POINT ( 'NONE',  ( -9.608651860293715430, 184.6439102242405284, 305.3492338956228309 ) ) ;
#13103=CARTESIAN_POINT ( 'NONE',  ( 12.18267571817558981, 187.8048479060753948, 322.6837437219421076 ) ) ;
#13116=CYLINDRICAL_SURFACE ( 'NONE', #19508, 22.50000000000000000 ) ;
#13131=DIRECTION ( 'NONE',  ( -0.5439613279325644646, -0.8390293148633950482, 0.01165686551792462916 ) ) ;
#13133=ORIENTED_EDGE ( 'NONE', *, *, #20639, .T. ) ;
#13134=CARTESIAN_POINT ( 'NONE',  ( 12.84376896873858875, 190.4863203672247494, 307.8501947603993472 ) ) ;
#13154=CARTESIAN_POINT ( 'NONE',  ( 17.97637993448925542, 184.5224678489072119, 318.9840103354205780 ) ) ;
#13175=EDGE_CURVE ( 'NONE', #18739, #17190, #14481, .T. ) ;
#13179=VERTEX_POINT ( 'NONE', #7540 ) ;
#13186=CARTESIAN_POINT ( 'NONE',  ( -8.348562176644710675, 185.3620174482674088, 323.2531432398233164 ) ) ;
#13191=EDGE_LOOP ( 'NONE', ( #2122, #14050 ) ) ;
#13193=CARTESIAN_POINT ( 'NONE',  ( -8.921762758010784111, 185.1413007774065989, 305.2050614739068237 ) ) ;
#13200=LINE ( 'NONE', #18152, #16285 ) ;
#13207=CARTESIAN_POINT ( 'NONE',  ( -15.41639432518098829, 177.9592009253594256, 316.4977043549463929 ) ) ;
#13218=EDGE_CURVE ( 'NONE', #17682, #5010, #14800, .T. ) ;
#13228=CARTESIAN_POINT ( 'NONE',  ( 16.39634482804422433, 187.9401017119210451, 319.7988598509798521 ) ) ;
#13229=CARTESIAN_POINT ( 'NONE',  ( 4.169604791867612015, 166.7785703876306513, 322.5944574396354483 ) ) ;
#13269=CARTESIAN_POINT ( 'NONE',  ( 19.48840479045136576, 184.2293629865677929, 316.4953788918857640 ) ) ;
#13313=CARTESIAN_POINT ( 'NONE',  ( -12.64734457064410478, 181.8784574882332379, 309.2558995593432769 ) ) ;
#13328=CARTESIAN_POINT ( 'NONE',  ( -13.52157056713759786, 180.8428797338423806, 308.0663627464555248 ) ) ;
#13337=CARTESIAN_POINT ( 'NONE',  ( -9.888959084247115783, 187.7288727309014860, 308.1497221693155097 ) ) ;
#13347=CARTESIAN_POINT ( 'NONE',  ( 13.05740731942213095, 190.2969143928351059, 320.8495709388896557 ) ) ;
#13389=CARTESIAN_POINT ( 'NONE',  ( 19.91815129952728469, 182.7044225173947893, 313.0591062094031258 ) ) ;
#13392=VECTOR ( 'NONE', #4523, 1000.000000000000114 ) ;
#13398=CARTESIAN_POINT ( 'NONE',  ( -10.85283309178001687, 186.7056505379215139, 320.9993531894351122 ) ) ;
#13399=ORIENTED_EDGE ( 'NONE', *, *, #5863, .T. ) ;
#13400=AXIS2_PLACEMENT_3D ( 'NONE', #19260, #20752, #5006 ) ;
#13405=ORIENTED_EDGE ( 'NONE', *, *, #18930, .T. ) ;
#13422=CARTESIAN_POINT ( 'NONE',  ( -12.18818533274768967, 185.3912375219357500, 308.8328755857670558 ) ) ;
#13423=ORIENTED_EDGE ( 'NONE', *, *, #15008, .T. ) ;
#13430=FACE_BOUND ( 'NONE', #17268, .T. ) ;
#13434=CARTESIAN_POINT ( 'NONE',  ( -14.50562271935455172, 179.3719498139292341, 319.5410565726744494 ) ) ;
#13444=CARTESIAN_POINT ( 'NONE',  ( -24.25006591444867965, 324.5132455039467345, 307.8723024395048355 ) ) ;
#13470=VERTEX_POINT ( 'NONE', #18302 ) ;
#13472=ORIENTED_EDGE ( 'NONE', *, *, #2190, .T. ) ;
#13490=ADVANCED_BREP_SHAPE_REPRESENTATION ( '', ( #17529, #6292 ), #18057 ) ;
#13519=EDGE_LOOP ( 'NONE', ( #3658, #7008, #6920, #5423 ) ) ;
#13534=CARTESIAN_POINT ( 'NONE',  ( -9.804288294571927409, 187.7022783261437837, 321.1616740932373091 ) ) ;
#13536=DIRECTION ( 'NONE',  ( 0.01292394549866727853, 0.005513023399720741458, 0.9999012842304692006 ) ) ;
#13547=CARTESIAN_POINT ( 'NONE',  ( -28.36560386230606667, 324.0744542294598887, 315.7670840739926916 ) ) ;
#13556=CARTESIAN_POINT ( 'NONE',  ( 14.26054767869631945, 189.5762264811534692, 320.6589299877209669 ) ) ;
#13603=CARTESIAN_POINT ( 'NONE',  ( 4.150218873619610171, 166.7703008525310793, 321.0946055132897072 ) ) ;
#13615=ORIENTED_EDGE ( 'NONE', *, *, #16410, .F. ) ;
#13628=CARTESIAN_POINT ( 'NONE',  ( 16.40873467035000033, 185.6567299720572635, 322.3321779654820602 ) ) ;
#13629=CARTESIAN_POINT ( 'NONE',  ( 13.03253886790000315, 190.3482298048060386, 320.8504275187944472 ) ) ;
#13652=CARTESIAN_POINT ( 'NONE',  ( 12.84540398394166871, 188.0649948051286344, 320.9599377868520378 ) ) ;
#13663=ORIENTED_EDGE ( 'NONE', *, *, #5816, .F. ) ;
#13664=CARTESIAN_POINT ( 'NONE',  ( 4.195452682864946325, 166.7895964344300808, 324.5942600080963985 ) ) ;
#13688=ORIENTED_EDGE ( 'NONE', *, *, #6726, .F. ) ;
#13714=VERTEX_POINT ( 'NONE', #12047 ) ;
#13727=CARTESIAN_POINT ( 'NONE',  ( -9.829296516163982034, 187.6860858752735908, 321.1599732488574546 ) ) ;
#13752=CARTESIAN_POINT ( 'NONE',  ( -9.979532414892725356, 187.9007632834477306, 308.1559136815830016 ) ) ;
#13763=FACE_OUTER_BOUND ( 'NONE', #21091, .T. ) ;
#13765=CARTESIAN_POINT ( 'NONE',  ( 13.32375866196222347, 190.1420591301118748, 320.8223493350537865 ) ) ;
#13769=DIRECTION ( 'NONE',  ( 0.3101392564284313202, 0.9506461370142480494, -0.009250070373107143265 ) ) ;
#13771=DIRECTION ( 'NONE',  ( 0.6295830517327242193, 0.6486237524303245516, 0.4276826028190943152 ) ) ;
#13773=DIRECTION ( 'NONE',  ( -0.01292394549866727679, -0.005513023399720743192, -0.9999012842304693116 ) ) ;
#13791=DIRECTION ( 'NONE',  ( 0.9934404589540163366, 0.1135548637187043797, -0.01346653032742958257 ) ) ;
#13811=DIRECTION ( 'NONE',  ( 0.1136178953597579561, -0.9935164314186356593, 0.004009283626633661397 ) ) ;
#13863=CARTESIAN_POINT ( 'NONE',  ( 0.3234033260118191477, 327.3504727214124728, 314.5682625988872587 ) ) ;
#13903=DIRECTION ( 'NONE',  ( -0.9999164797902017066, 0.000000000000000000, 0.01292414190463972781 ) ) ;
#13908=ADVANCED_FACE ( 'NONE', ( #3345 ), #12207, .F. ) ;
#13909=ORIENTED_EDGE ( 'NONE', *, *, #11346, .T. ) ;
#13910=CARTESIAN_POINT ( 'NONE',  ( 21.64049994983132663, 168.7353503906255412, 312.3898283681904786 ) ) ;
#13933=CARTESIAN_POINT ( 'NONE',  ( -12.09763426542455811, 164.9045537938005452, 319.1981365539348872 ) ) ;
#13945=CIRCLE ( 'NONE', #5110, 8.520833333333293069 ) ;
#13962=EDGE_CURVE ( 'NONE', #11132, #4095, #20685, .T. ) ;
#13977=CARTESIAN_POINT ( 'NONE',  ( -9.829281886977605964, 187.6860989516580389, 321.1599752159536365 ) ) ;
#13979=ADVANCED_FACE ( 'NONE', ( #15771 ), #3826, .F. ) ;
#13982=CARTESIAN_POINT ( 'NONE',  ( 12.23383248052724070, 187.6909830581990946, 322.9726054647817364 ) ) ;
#14009=EDGE_CURVE ( 'NONE', #3703, #11287, #10024, .T. ) ;
#14012=DIRECTION ( 'NONE',  ( 0.01292394549866727679, 0.005513023399720742325, 0.9999012842304692006 ) ) ;
#14025=EDGE_LOOP ( 'NONE', ( #5606, #3926, #21376, #20314, #16319, #13472, #5887, #3260, #12611, #7836 ) ) ;
#14040=CARTESIAN_POINT ( 'NONE',  ( 19.92486830831109046, 168.5282407225510326, 309.6860031901712205 ) ) ;
#14050=ORIENTED_EDGE ( 'NONE', *, *, #15024, .T. ) ;
#14052=AXIS2_PLACEMENT_3D ( 'NONE', #22551, #3516, #305 ) ;
#14061=CARTESIAN_POINT ( 'NONE',  ( -28.05907253792918610, 324.1127586016892224, 316.5723599207789789 ) ) ;
#14076=CARTESIAN_POINT ( 'NONE',  ( 17.35534499068185710, 186.7833359346272175, 309.5258091127471971 ) ) ;
#14081=EDGE_CURVE ( 'NONE', #21571, #5484, #20876, .T. ) ;
#14086=( LENGTH_UNIT ( ) NAMED_UNIT ( * ) SI_UNIT ( .MILLI., .METRE. ) );
#14088=CARTESIAN_POINT ( 'NONE',  ( 20.29114497646528648, 182.2714854321924918, 311.7131426610552012 ) ) ;
#14103=DIRECTION ( 'NONE',  ( -0.01292394549866745720, -0.005513023399720816918, -0.9999012842304692006 ) ) ;
#14115=CARTESIAN_POINT ( 'NONE',  ( -9.899470319389305217, 187.6214926260726656, 321.1548253226370093 ) ) ;
#14119=CARTESIAN_POINT ( 'NONE',  ( -15.15257079676713126, 179.5546631012716432, 315.4103692381972905 ) ) ;
#14123=CARTESIAN_POINT ( 'NONE',  ( 15.86053680860744564, 168.0563658420342961, 307.9314113524436038 ) ) ;
#14124=CARTESIAN_POINT ( 'NONE',  ( -15.04605271383937470, 179.9046364190501208, 313.1717202347408033 ) ) ;
#14126=CARTESIAN_POINT ( 'NONE',  ( 20.56772423864910948, 182.0615390744364106, 316.0167400927113590 ) ) ;
#14137=DIRECTION ( 'NONE',  ( -0.9506032891036972909, 0.3102281881984321754, 0.01057629388542893900 ) ) ;
#14155=DIRECTION ( 'NONE',  ( 0.1351880940536942799, -0.9908129862407182298, 0.003715578404455081168 ) ) ;
#14156=CARTESIAN_POINT ( 'NONE',  ( 16.07150438106780399, 168.1329592171555305, 320.9330071493605487 ) ) ;
#14168=EDGE_CURVE ( 'NONE', #11287, #18203, #8584, .T. ) ;
#14178=CARTESIAN_POINT ( 'NONE',  ( -27.71828981744229381, 324.1286477571945284, 310.8524157770490888 ) ) ;
#14202=DIRECTION ( 'NONE',  ( -0.01292394549866745720, -0.005513023399720816918, -0.9999012842304692006 ) ) ;
#14204=FILL_AREA_STYLE ('',( #10399 ) ) ;
#14206=CARTESIAN_POINT ( 'NONE',  ( 13.11950053790673998, 190.3195187405954130, 307.8718610784719658 ) ) ;
#14230=CARTESIAN_POINT ( 'NONE',  ( -10.25967351461796362, 187.2843258730522393, 321.1153754285980426 ) ) ;
#14234=CARTESIAN_POINT ( 'NONE',  ( -10.02117361870881851, 187.8727420016839176, 308.1601407300097435 ) ) ;
#14237=CARTESIAN_POINT ( 'NONE',  ( 16.44044660180618678, 168.1228407995204179, 307.9702792283749773 ) ) ;
#14238=CARTESIAN_POINT ( 'NONE',  ( -14.25139930150079515, 179.7940826540526871, 318.1440894004308007 ) ) ;
#14239=CARTESIAN_POINT ( 'NONE',  ( 17.86254487970774463, 184.6173340417515760, 321.1453017134867309 ) ) ;
#14263=CARTESIAN_POINT ( 'NONE',  ( -3.492210504507778257, 326.9352113893252749, 319.7943972700559243 ) ) ;
#14276=ORIENTED_EDGE ( 'NONE', *, *, #9579, .T. ) ;
#14283=CARTESIAN_POINT ( 'NONE',  ( -27.47457004210972897, 324.1549168750700574, 310.4553055122309502 ) ) ;
#14302=CARTESIAN_POINT ( 'NONE',  ( 19.75650998535411063, 183.7491368459512842, 312.9879496513954678 ) ) ;
#14318=CARTESIAN_POINT ( 'NONE',  ( 16.09649071154515099, 185.6410692198624020, 306.2537067563579285 ) ) ;
#14324=CARTESIAN_POINT ( 'NONE',  ( -8.637836329777936584, 185.8852932021121376, 322.1857653656461480 ) ) ;
#14329=ORIENTED_EDGE ( 'NONE', *, *, #19877, .F. ) ;
#14351=CARTESIAN_POINT ( 'NONE',  ( -15.03108941308168234, 179.9501653168765358, 313.0619997550173252 ) ) ;
#14354=EDGE_LOOP ( 'NONE', ( #18576, #1974, #3834, #7330 ) ) ;
#14356=CARTESIAN_POINT ( 'NONE',  ( -13.20095895536456609, 181.0966850513278814, 321.5989609326452978 ) ) ;
#14375=CARTESIAN_POINT ( 'NONE',  ( -5.703700719415883746, 174.2634384100414593, 299.6785330862965679 ) ) ;
#14376=EDGE_LOOP ( 'NONE', ( #7211, #7041, #11700, #6032, #13423 ) ) ;
#14377=ORIENTED_EDGE ( 'NONE', *, *, #13218, .T. ) ;
#14394=AXIS2_PLACEMENT_3D ( 'NONE', #360, #15895, #10698 ) ;
#14410=CARTESIAN_POINT ( 'NONE',  ( -8.308020146049644339, 165.3460916013453641, 321.2202151032084316 ) ) ;
#14424=CARTESIAN_POINT ( 'NONE',  ( 19.80241179164982768, 183.7441055747629264, 315.5604959055339691 ) ) ;
#14425=AXIS2_PLACEMENT_3D ( 'NONE', #11438, #2714, #7975 ) ;
#14431=EDGE_CURVE ( 'NONE', #7715, #18203, #16503, .T. ) ;
#14435=EDGE_CURVE ( 'NONE', #3953, #19042, #8259, .T. ) ;
#14439=CARTESIAN_POINT ( 'NONE',  ( 12.90652684605866796, 190.4489680158945646, 307.8543765190132717 ) ) ;
#14443=( BOUNDED_SURFACE ( )  B_SPLINE_SURFACE ( 3, 2, ( 
 ( #17300, #15587, #20176 ),
 ( #1560, #22000, #18584 ),
 ( #8546, #8652, #7904 ),
 ( #11473, #15695, #18479 ),
 ( #16876, #19231, #14941 ),
 ( #12123, #22535, #22636 ),
 ( #6827, #9754, #3385 ),
 ( #6301, #11588, #20830 ),
 ( #10401, #1678, #6933 ),
 ( #5211, #12244, #3500 ),
 ( #16663, #5666, #14439 ),
 ( #14546, #5325, #5434 ),
 ( #17883, #10515, #14206 ),
 ( #12467, #8888, #17640 ),
 ( #2225, #9002, #2115 ),
 ( #17527, #19779, #1780 ),
 ( #10617, #19455, #10961 ),
 ( #17987, #3604, #181 ),
 ( #21072, #9109, #3721 ),
 ( #14318, #12364, #21400 ),
 ( #1896, #8757, #21505 ),
 ( #21180, #21285, #15933 ),
 ( #9231, #12703, #15811 ),
 ( #7176, #10741, #5771 ),
 ( #19670, #7278, #16278 ),
 ( #17769, #19345, #3940 ),
 ( #55, #2013, #16048 ),
 ( #283, #5556, #7058 ),
 ( #12586, #19569, #3844 ),
 ( #10858, #16159, #518 ),
 ( #12806, #399, #7395 ),
 ( #14088, #7518, #7619 ),
 ( #21946, #19902, #4172 ),
 ( #18545, #18213, #20016 ),
 ( #4053, #13389, #11081 ),
 ( #11199, #6018, #4510 ),
 ( #11540, #2458, #16492 ),
 ( #14661, #2697, #21731 ),
 ( #7859, #5897, #7960 ),
 ( #9455, #18105, #15110 ),
 ( #2348, #746, #6368 ),
 ( #2802, #6243, #9349 ),
 ( #7741, #4279, #14994 ),
 ( #18431, #11304, #13269 ),
 ( #9810, #16826, #13055 ),
 ( #16726, #18308, #21612 ),
 ( #16387, #9706, #14781 ),
 ( #2575, #12933, #628 ),
 ( #9584, #16618, #869 ),
 ( #14896, #21838, #6128 ),
 ( #20247, #13154, #20118 ),
 ( #11418, #4389, #974 ),
 ( #1083, #22066, #8075 ),
 ( #17393, #22615, #17271 ),
 ( #15562, #1208, #6580 ),
 ( #3020, #8203, #2907 ) ),
 .UNSPECIFIED., .F., .F., .T. ) 
 B_SPLINE_SURFACE_WITH_KNOTS ( ( 4, 2, 2, 2, 2, 2, 2, 2, 2, 2, 2, 2, 2, 2, 2, 2, 2, 2, 2, 2, 2, 2, 2, 2, 2, 2, 2, 4 ),
 ( 3, 3 ),
 ( 0.1242173993009022120, 0.1244328327546842528, 0.1244866911181297664, 0.1245136202998525232, 0.1245405494815752800, 0.1246482662084663073, 0.1250791331160303888, 0.1259408669311585793, 0.1276643345614149605, 0.1293878021916713417, 0.1311112698219276951, 0.1328347374521840485, 0.1345582050824404297, 0.1362816727126968108, 0.1371434065278249737, 0.1380051403429531642, 0.1388668741580813548, 0.1397286079732095176, 0.1405903417883377082, 0.1414520756034658988, 0.1431755432337222800, 0.1440372770488504706, 0.1448990108639786611, 0.1457607446791068517, 0.1466224784942350423, 0.1483459461244913957, 0.1500694137547477491, 0.1517928813850041303 ),
 ( 0.000000000000000000, 1.000000000000000000 ),
 .UNSPECIFIED. ) 
 GEOMETRIC_REPRESENTATION_ITEM ( )  RATIONAL_B_SPLINE_SURFACE ( (
 ( 1.000000000000000000, 0.7202457815375945538, 1.000000000000000000),
 ( 1.000000000000000000, 0.7203148644494854480, 1.000000000000000000),
 ( 1.000000000000000000, 0.7203837616398036658, 1.000000000000000000),
 ( 1.000000000000000000, 0.7204696515171350457, 1.000000000000000000),
 ( 1.000000000000000000, 0.7204868179141954432, 1.000000000000000000),
 ( 1.000000000000000000, 0.7205125501470087679, 1.000000000000000000),
 ( 1.000000000000000000, 0.7205211246666077818, 1.000000000000000000),
 ( 1.000000000000000000, 0.7205382679145281299, 1.000000000000000000),
 ( 1.000000000000000000, 0.7207549634841317054, 1.000000000000000000),
 ( 1.000000000000000000, 0.7214802973574021561, 1.000000000000000000),
 ( 1.000000000000000000, 0.7220635808725176519, 1.000000000000000000),
 ( 1.000000000000000000, 0.7249944760233909546, 1.000000000000000000),
 ( 1.000000000000000000, 0.7273854792137299796, 1.000000000000000000),
 ( 1.000000000000000000, 0.7346752236034637118, 1.000000000000000000),
 ( 1.000000000000000000, 0.7396903655602768968, 1.000000000000000000),
 ( 1.000000000000000000, 0.7550399040982476162, 1.000000000000000000),
 ( 1.000000000000000000, 0.7655727772217874039, 1.000000000000000000),
 ( 1.000000000000000000, 0.7871107331848644639, 1.000000000000000000),
 ( 1.000000000000000000, 0.7981416010053231647, 1.000000000000000000),
 ( 1.000000000000000000, 0.8197093954368291913, 1.000000000000000000),
 ( 1.000000000000000000, 0.8303367115343781579, 1.000000000000000000),
 ( 1.000000000000000000, 0.8510544108449787926, 1.000000000000000000),
 ( 1.000000000000000000, 0.8611795848883848636, 1.000000000000000000),
 ( 1.000000000000000000, 0.8805664355309501534, 1.000000000000000000),
 ( 1.000000000000000000, 0.8897650402490725474, 1.000000000000000000),
 ( 1.000000000000000000, 0.9068567199018958691, 1.000000000000000000),
 ( 1.000000000000000000, 0.9147565445290845032, 1.000000000000000000),
 ( 1.000000000000000000, 0.9255566967665967981, 1.000000000000000000),
 ( 1.000000000000000000, 0.9289711410761075649, 1.000000000000000000),
 ( 1.000000000000000000, 0.9352102042489658373, 1.000000000000000000),
 ( 1.000000000000000000, 0.9380652775089347584, 1.000000000000000000),
 ( 1.000000000000000000, 0.9432152439419067003, 1.000000000000000000),
 ( 1.000000000000000000, 0.9455148386610635614, 1.000000000000000000),
 ( 1.000000000000000000, 0.9494488520115715868, 1.000000000000000000),
 ( 1.000000000000000000, 0.9510350116254054909, 1.000000000000000000),
 ( 1.000000000000000000, 0.9534119305046732107, 1.000000000000000000),
 ( 1.000000000000000000, 0.9542080638533945169, 1.000000000000000000),
 ( 1.000000000000000000, 0.9549528115835310693, 1.000000000000000000),
 ( 1.000000000000000000, 0.9548852033311120424, 1.000000000000000000),
 ( 1.000000000000000000, 0.9533785252478389483, 1.000000000000000000),
 ( 1.000000000000000000, 0.9507260831990033134, 1.000000000000000000),
 ( 1.000000000000000000, 0.9445325143455129968, 1.000000000000000000),
 ( 1.000000000000000000, 0.9421267862709985508, 1.000000000000000000),
 ( 1.000000000000000000, 0.9368091832047875656, 1.000000000000000000),
 ( 1.000000000000000000, 0.9338841920341318659, 1.000000000000000000),
 ( 1.000000000000000000, 0.9275336217117351456, 1.000000000000000000),
 ( 1.000000000000000000, 0.9240930730323024811, 1.000000000000000000),
 ( 1.000000000000000000, 0.9167918297806771921, 1.000000000000000000),
 ( 1.000000000000000000, 0.9129208614828339119, 1.000000000000000000),
 ( 1.000000000000000000, 0.9008886848957327054, 1.000000000000000000),
 ( 1.000000000000000000, 0.8922078542948799207, 1.000000000000000000),
 ( 1.000000000000000000, 0.8738477936028254955, 1.000000000000000000),
 ( 1.000000000000000000, 0.8641886109620656731, 1.000000000000000000),
 ( 1.000000000000000000, 0.8438841653332657122, 1.000000000000000000),
 ( 1.000000000000000000, 0.8333285471625734298, 1.000000000000000000),
 ( 1.000000000000000000, 0.8227386401547407413, 1.000000000000000000) ) ) 
 REPRESENTATION_ITEM ( '' )  SURFACE ( )  );
#14477=CARTESIAN_POINT ( 'NONE',  ( -15.55314327042932376, 177.7443265726918469, 314.9881042928857369 ) ) ;
#14481=CIRCLE ( 'NONE', #18488, 10.29357798165139393 ) ;
#14500=ORIENTED_EDGE ( 'NONE', *, *, #27, .T. ) ;
#14505=ORIENTED_EDGE ( 'NONE', *, *, #12257, .T. ) ;
#14520=CARTESIAN_POINT ( 'NONE',  ( -12.81536461602102683, 326.2504838843369726, 414.3222871145668478 ) ) ;
#14523=CARTESIAN_POINT ( 'NONE',  ( -22.57586261656929238, 324.7034503240921026, 307.5610645536022503 ) ) ;
#14535=CARTESIAN_POINT ( 'NONE',  ( 19.56521222682726702, 184.0192530622549043, 312.4160503478434521 ) ) ;
#14543=CARTESIAN_POINT ( 'NONE',  ( -10.03308090247307405, 188.0016273849522861, 308.1595840160059083 ) ) ;
#14546=CARTESIAN_POINT ( 'NONE',  ( 12.19776044723496256, 187.6128494603106276, 304.9050912290015276 ) ) ;
#14569=( BOUNDED_SURFACE ( )  B_SPLINE_SURFACE ( 3, 2, ( 
 ( #19259, #19481, #3631 ),
 ( #1805, #3756, #12497 ),
 ( #10769, #3525, #20979 ),
 ( #5232, #7429, #10879 ),
 ( #8790, #2139, #12275 ),
 ( #15844, #9139, #16191 ),
 ( #14230, #431, #10537 ),
 ( #313, #21434, #8914 ),
 ( #7305, #87, #5696 ),
 ( #14115, #10644, #17679 ),
 ( #1927, #203, #15964 ),
 ( #21204, #11568, #9738 ),
 ( #11449, #9617, #5926 ),
 ( #15026, #4081, #6161 ),
 ( #7548, #11228, #7886 ),
 ( #7642, #20048, #13186 ),
 ( #16647, #658, #4305 ),
 ( #19930, #20152, #14576 ) ),
 .UNSPECIFIED., .F., .F., .T. ) 
 B_SPLINE_SURFACE_WITH_KNOTS ( ( 4, 2, 2, 2, 2, 2, 2, 2, 4 ),
 ( 3, 3 ),
 ( 0.08392082777186243847, 0.08669808355430655422, 0.08808671144552862597, 0.08878102539113966185, 0.08912818236394517979, 0.08930176085034793876, 0.08934515547194862850, 0.08938855009354931824, 0.08947533933675068385 ),
 ( 0.000000000000000000, 1.000000000000000000 ),
 .UNSPECIFIED. ) 
 GEOMETRIC_REPRESENTATION_ITEM ( )  RATIONAL_B_SPLINE_SURFACE ( (
 ( 1.000000000000000000, 0.8227386401548728578, 1.000000000000000000),
 ( 1.000000000000000000, 0.8263415838687132586, 1.000000000000000000),
 ( 1.000000000000000000, 0.8288608359724080055, 1.000000000000000000),
 ( 1.000000000000000000, 0.8282189721166841601, 1.000000000000000000),
 ( 1.000000000000000000, 0.8271574078635184346, 1.000000000000000000),
 ( 1.000000000000000000, 0.8239197622700882295, 1.000000000000000000),
 ( 1.000000000000000000, 0.8225730560414692416, 1.000000000000000000),
 ( 1.000000000000000000, 0.8201245374459615878, 1.000000000000000000),
 ( 1.000000000000000000, 0.8192370252863434565, 1.000000000000000000),
 ( 1.000000000000000000, 0.8177961922883111301, 1.000000000000000000),
 ( 1.000000000000000000, 0.8172976608660983411, 1.000000000000000000),
 ( 1.000000000000000000, 0.8166514735310177464, 1.000000000000000000),
 ( 1.000000000000000000, 0.8167936669037794140, 1.000000000000000000),
 ( 1.000000000000000000, 0.8168953424636213878, 1.000000000000000000),
 ( 1.000000000000000000, 0.8169461963287523165, 1.000000000000000000),
 ( 1.000000000000000000, 0.8170988061681787595, 1.000000000000000000),
 ( 1.000000000000000000, 0.8172006103753840511, 1.000000000000000000),
 ( 1.000000000000000000, 0.8173024788409735120, 1.000000000000000000) ) ) 
 REPRESENTATION_ITEM ( '' )  SURFACE ( )  );
#14576=CARTESIAN_POINT ( 'NONE',  ( -8.305185890944088101, 185.3905336583419512, 323.2540923045081058 ) ) ;
#14580=CARTESIAN_POINT ( 'NONE',  ( -12.58664483627419095, 184.6272112293399630, 320.1917372557430213 ) ) ;
#14582=CARTESIAN_POINT ( 'NONE',  ( -14.97537071516516427, 178.7788208869449136, 313.2939786621885787 ) ) ;
#14587=EDGE_CURVE ( 'NONE', #20005, #126, #16708, .T. ) ;
#14605=CARTESIAN_POINT ( 'NONE',  ( 12.53551711061738594, 188.9428922227077976, 321.3016085981989818 ) ) ;
#14627=EDGE_CURVE ( 'NONE', #17067, #19550, #15117, .T. ) ;
#14641=CARTESIAN_POINT ( 'NONE',  ( 12.84375058515307089, 190.4863273772031960, 307.8501935766865927 ) ) ;
#14646=CARTESIAN_POINT ( 'NONE',  ( 13.21943290499836543, 190.2582281869503049, 307.8807104300166202 ) ) ;
#14661=CARTESIAN_POINT ( 'NONE',  ( 20.69718713607370475, 181.8844827137008053, 314.2148154440831718 ) ) ;
#14670=ORIENTED_EDGE ( 'NONE', *, *, #6988, .F. ) ;
#14692=ORIENTED_EDGE ( 'NONE', *, *, #7534, .T. ) ;
#14695=CARTESIAN_POINT ( 'NONE',  ( -14.88208367441968072, 180.3442769117117166, 312.4626966567733461 ) ) ;
#14706=AXIS2_PLACEMENT_3D ( 'NONE', #8458, #15506, #12159 ) ;
#14724=CARTESIAN_POINT ( 'NONE',  ( 19.87979702288915718, 182.8092583941872533, 318.2062520007012267 ) ) ;
#14750=ORIENTED_EDGE ( 'NONE', *, *, #1370, .F. ) ;
#14781=CARTESIAN_POINT ( 'NONE',  ( 19.15828809225966722, 184.7089495515359943, 317.1432155856761028 ) ) ;
#14790=CARTESIAN_POINT ( 'NONE',  ( -22.66159625276162970, 324.6936785073799001, 307.5691494985305781 ) ) ;
#14800=LINE ( 'NONE', #11103, #3424 ) ;
#14805=CARTESIAN_POINT ( 'NONE',  ( -19.28847592064633787, 309.3375565838056787, 328.6122914246403184 ) ) ;
#14815=CARTESIAN_POINT ( 'NONE',  ( -10.63046908155944692, 187.2581710861182671, 308.2567892644384528 ) ) ;
#14817=ORIENTED_EDGE ( 'NONE', *, *, #2190, .F. ) ;
#14829=CARTESIAN_POINT ( 'NONE',  ( -11.36765543714179394, 183.1705039132345973, 306.0958062668278785 ) ) ;
#14835=AXIS2_PLACEMENT_3D ( 'NONE', #1775, #14202, #19566 ) ;
#14861=ORIENTED_EDGE ( 'NONE', *, *, #6425, .T. ) ;
#14882=AXIS2_PLACEMENT_3D ( 'NONE', #8634, #19322, #10263 ) ;
#14896=CARTESIAN_POINT ( 'NONE',  ( 19.03050207494622725, 183.6302965638845137, 319.7390526622639300 ) ) ;
#14932=CARTESIAN_POINT ( 'NONE',  ( -13.76919743346306646, 180.5356774100213784, 310.4380730639882131 ) ) ;
#14936=CARTESIAN_POINT ( 'NONE',  ( 12.55221694283142853, 189.7895332285891641, 307.7358867228051622 ) ) ;
#14941=CARTESIAN_POINT ( 'NONE',  ( 12.79778896233726471, 190.5038093453642603, 307.8472338899999841 ) ) ;
#14942=CARTESIAN_POINT ( 'NONE',  ( -13.22370634329071848, 181.0695397079195459, 321.5726873589048864 ) ) ;
#14950=CARTESIAN_POINT ( 'NONE',  ( -9.296350947641979445, 186.8092295296417262, 307.8158422510384185 ) ) ;
#14994=CARTESIAN_POINT ( 'NONE',  ( 19.62580668441758647, 184.0217288607373121, 316.1492713539591364 ) ) ;
#15008=EDGE_CURVE ( 'NONE', #2643, #8739, #17318, .T. ) ;
#15024=EDGE_CURVE ( 'NONE', #17822, #18942, #4100, .T. ) ;
#15026=CARTESIAN_POINT ( 'NONE',  ( -9.786139105534834570, 187.7140077023060485, 321.1629084044704996 ) ) ;
#15033=CARTESIAN_POINT ( 'NONE',  ( -11.49837594199064839, 183.0688075479256440, 306.1363948905710117 ) ) ;
#15037=SHAPE_REPRESENTATION ( 'Handle Handwheel Knob', ( #6292 ), #18057 ) ;
#15045=CARTESIAN_POINT ( 'NONE',  ( -15.51054658338874326, 177.8073622993804861, 315.7124409163076280 ) ) ;
#15054=CIRCLE ( 'NONE', #10346, 2.999999999999994227 ) ;
#15067=CARTESIAN_POINT ( 'NONE',  ( 26.54786300933031740, 169.3445808681009623, 324.2912630757292050 ) ) ;
#15073=( GEOMETRIC_REPRESENTATION_CONTEXT ( 3 ) GLOBAL_UNCERTAINTY_ASSIGNED_CONTEXT ( ( #5540 ) ) GLOBAL_UNIT_ASSIGNED_CONTEXT ( ( #14086, #1675, #15693 ) ) REPRESENTATION_CONTEXT ( 'NONE', 'WORKASPACE' ) );
#15110=CARTESIAN_POINT ( 'NONE',  ( 19.91008402892363094, 183.5677589090103652, 315.0360073274616752 ) ) ;
#15117=B_SPLINE_CURVE_WITH_KNOTS ( 'NONE', 3,
 ( #3928, #12352, #10948, #2213, #7380, #10726, #9094, #7265, #3593, #385, #504, #8744, #14424, #8990, #273, #7507, #10603, #5314, #21057, #17628, #14302, #21271, #14535, #5196, #12234, #3490, #10506, #17517, #14076, #7046, #15800, #41, #1882, #166, #7163, #7850, #730, #14646, #21720, #19766 ),
 .UNSPECIFIED., .F., .F.,
 ( 4, 2, 2, 2, 2, 2, 2, 2, 2, 2, 2, 2, 2, 2, 2, 2, 2, 2, 2, 4 ),
 ( 0.004439741376687713660, 0.005757347133595717287, 0.007074952890503720046, 0.008392558647411722805, 0.009710164404319727299, 0.01102777016122773006, 0.01168657303968165945, 0.01234537591813558710, 0.01300417879658951822, 0.01366298167504344588, 0.01432178455349737700, 0.01498058743195130466, 0.01629819318885934037, 0.01761579894576737609, 0.02025101045958349263, 0.02156861621649154917, 0.02288622197339960918, 0.02420382773030766571, 0.02486263060876169745, 0.02552143348721572919 ),
 .UNSPECIFIED. ) ;
#15153=CARTESIAN_POINT ( 'NONE',  ( -14.74258221042073913, 179.1459434199334169, 310.2631537442956642 ) ) ;
#15237=EDGE_CURVE ( 'NONE', #17518, #21242, #2504, .T. ) ;
#15267=CARTESIAN_POINT ( 'NONE',  ( -10.24828629132402824, 187.6512746430315985, 308.1882031990034534 ) ) ;
#15279=DIRECTION ( 'NONE',  ( 0.9934404589540163366, 0.1135548637187057258, -0.01346653032743021922 ) ) ;
#15298=ORIENTED_EDGE ( 'NONE', *, *, #21487, .F. ) ;
#15314=LINE ( 'NONE', #8171, #18347 ) ;
#15318=VERTEX_POINT ( 'NONE', #22652 ) ;
#15325=ORIENTED_EDGE ( 'NONE', *, *, #3510, .F. ) ;
#15326=EDGE_CURVE ( 'NONE', #5010, #6442, #12865, .T. ) ;
#15351=VERTEX_POINT ( 'NONE', #4995 ) ;
#15362=CARTESIAN_POINT ( 'NONE',  ( 13.02962957137955335, 190.4272972286120478, 320.8494027134000817 ) ) ;
#15364=DIRECTION ( 'NONE',  ( 0.01292394549866742078, 0.005513023399720777019, 0.9999012842304693116 ) ) ;
#15381=CARTESIAN_POINT ( 'NONE',  ( -9.820930688317483614, 187.6915098723768267, 321.1605422340256837 ) ) ;
#15390=CARTESIAN_POINT ( 'NONE',  ( 12.16442896649338223, 187.7168230983759543, 322.9757373289252200 ) ) ;
#15431=VERTEX_POINT ( 'NONE', #642 ) ;
#15465=ORIENTED_EDGE ( 'NONE', *, *, #220, .F. ) ;
#15474=CARTESIAN_POINT ( 'NONE',  ( 12.83169261137808981, 190.5749574533797954, 307.8498635260945662 ) ) ;
#15495=CARTESIAN_POINT ( 'NONE',  ( -4.928638145297007611, 326.7208992129484955, 307.3934828099208403 ) ) ;
#15506=DIRECTION ( 'NONE',  ( -0.01292394549866741904, -0.005513023399720750131, -0.9999012842304692006 ) ) ;
#15510=CARTESIAN_POINT ( 'NONE',  ( 18.76359067764538935, 183.6785240391465948, 308.7090574097932176 ) ) ;
#15513=TOROIDAL_SURFACE ( 'NONE', #14425, 20.50000000000000355, 2.000000000000000000 ) ;
#15529=DIRECTION ( 'NONE',  ( -0.01292394549866745720, -0.005513023399720816918, -0.9999012842304692006 ) ) ;
#15546=ORIENTED_EDGE ( 'NONE', *, *, #7534, .F. ) ;
#15559=ORIENTED_EDGE ( 'NONE', *, *, #18322, .T. ) ;
#15562=CARTESIAN_POINT ( 'NONE',  ( 16.78462010304006924, 185.4095063563936492, 322.0781884391542462 ) ) ;
#15567=CIRCLE ( 'NONE', #14835, 10.00000000000001421 ) ;
#15571=CARTESIAN_POINT ( 'NONE',  ( -12.22010268980495518, 185.1830022132863292, 320.4502402655688797 ) ) ;
#15587=CARTESIAN_POINT ( 'NONE',  ( 11.56915902040221944, 187.8794726123035730, 307.7516944564536630 ) ) ;
#15594=CARTESIAN_POINT ( 'NONE',  ( -8.586189643308495434, 185.3704654934846019, 305.1611493308044487 ) ) ;
#15598=B_SPLINE_CURVE_WITH_KNOTS ( 'NONE', 3,
 ( #14234, #21210, #17683, #19372, #18140, #3637, #12502, #318, #10774, #17805, #19486, #2041, #5700, #9026, #21098, #14351, #16078, #1931, #553, #2144, #7311, #14119, #9382, #12622, #19599, #2390, #662, #10991, #7552, #10650, #9143, #5353, #435, #3871, #16197, #14580 ),
 .UNSPECIFIED., .F., .F.,
 ( 4, 2, 2, 2, 2, 2, 2, 2, 2, 2, 2, 2, 2, 2, 2, 2, 2, 4 ),
 ( -5.999999999438343828E-08, 0.001317362229350502222, 0.002634784458700998883, 0.005269628917401928889, 0.006587051146752356812, 0.007904473376102786469, 0.009221895605453214392, 0.01053931783480364405, 0.01185674006415407197, 0.01251545117882927639, 0.01317416229350447908, 0.01383287340817968350, 0.01449158452285488619, 0.01580900675220515278, 0.01712642898155541590, 0.01844385121090567556, 0.01976127344025593868, 0.02107869566960620181 ),
 .UNSPECIFIED. ) ;
#15602=CARTESIAN_POINT ( 'NONE',  ( -2.015769147932460648, 327.0595725865082386, 308.7711644834471372 ) ) ;
#15622=CARTESIAN_POINT ( 'NONE',  ( 20.55752130627328000, 182.0093730182867944, 312.8173236010051141 ) ) ;
#15647=CARTESIAN_POINT ( 'NONE',  ( 13.44840881021241152, 159.0401032888326824, 299.5149227183727589 ) ) ;
#15650=ORIENTED_EDGE ( 'NONE', *, *, #11972, .T. ) ;
#15652=CARTESIAN_POINT ( 'NONE',  ( 19.10689234852680585, 168.4757078209644021, 319.8485184630963545 ) ) ;
#15660=FACE_OUTER_BOUND ( 'NONE', #10905, .T. ) ;
#15693=( NAMED_UNIT ( * ) SI_UNIT ( $, .STERADIAN. ) SOLID_ANGLE_UNIT ( ) );
#15695=CARTESIAN_POINT ( 'NONE',  ( 11.76425125167022578, 187.8086852021691016, 307.7642755247033506 ) ) ;
#15701=CARTESIAN_POINT ( 'NONE',  ( -12.81536461602102683, 326.2504838843369726, 414.3222871145668478 ) ) ;
#15702=CARTESIAN_POINT ( 'NONE',  ( -8.195910149518317311, 185.6194122973667788, 308.0197546130458477 ) ) ;
#15719=CARTESIAN_POINT ( 'NONE',  ( 12.99862026951066518, 190.3184116425491368, 320.8540507871223326 ) ) ;
#15724=CARTESIAN_POINT ( 'NONE',  ( 18.27202492469069028, 422.9831327814429756, 371.0727646550985241 ) ) ;
#15734=CARTESIAN_POINT ( 'NONE',  ( 20.66284806145036157, 181.9102389805751159, 313.6090225492346804 ) ) ;
#15763=CARTESIAN_POINT ( 'NONE',  ( -1.710339879361044035, 327.0957934528446458, 309.0913701133406448 ) ) ;
#15771=FACE_OUTER_BOUND ( 'NONE', #6000, .T. ) ;
#15779=CIRCLE ( 'NONE', #8059, 10.29357798165139393 ) ;
#15786=CARTESIAN_POINT ( 'NONE',  ( -10.97446589277025808, 164.9932245799013799, 309.3419758684869976 ) ) ;
#15800=CARTESIAN_POINT ( 'NONE',  ( 16.22504546523506264, 187.9132589410656919, 308.8173052943575954 ) ) ;
#15811=CARTESIAN_POINT ( 'NONE',  ( 17.35553945970433887, 186.7678997353801549, 309.5505051628369415 ) ) ;
#15842=CARTESIAN_POINT ( 'NONE',  ( 5.178247477726851677, 158.1956793026589025, 324.6289403114667493 ) ) ;
#15844=CARTESIAN_POINT ( 'NONE',  ( -10.38911361869056904, 187.1603952044747814, 321.0948210509291130 ) ) ;
#15848=CARTESIAN_POINT ( 'NONE',  ( -14.17380171632341224, 184.4915598789741011, 322.7338882641075770 ) ) ;
#15854=CARTESIAN_POINT ( 'NONE',  ( -14.58871019898540489, 179.2506784104788835, 319.3598715905317249 ) ) ;
#15859=DIRECTION ( 'NONE',  ( -0.01292394549866727679, -0.005513023399720743192, -0.9999012842304693116 ) ) ;
#15862=VECTOR ( 'NONE', #21348, 1000.000000000000227 ) ;
#15879=ORIENTED_EDGE ( 'NONE', *, *, #5675, .F. ) ;
#15895=DIRECTION ( 'NONE',  ( -0.3101392564284290998, -0.9506461370142487155, 0.009250070373107117244 ) ) ;
#15898=CARTESIAN_POINT ( 'NONE',  ( -4.397794363141794172, 165.8073523762867012, 324.7117453967128995 ) ) ;
#15901=ADVANCED_FACE ( 'NONE', ( #20987 ), #4997, .F. ) ;
#15908=CARTESIAN_POINT ( 'NONE',  ( -28.49296332856286185, 324.0493105597922749, 313.1455847166214426 ) ) ;
#15933=CARTESIAN_POINT ( 'NONE',  ( 17.07179474224462723, 187.0711841522102930, 309.3407821921324512 ) ) ;
#15945=CIRCLE ( 'NONE', #4896, 7.000000000000022204 ) ;
#15952=CARTESIAN_POINT ( 'NONE',  ( -13.92525281995234820, 325.7770340667113942, 328.4523304068723064 ) ) ;
#15957=CARTESIAN_POINT ( 'NONE',  ( 12.88848270841033639, 190.3578502642233445, 320.8635863820699115 ) ) ;
#15964=CARTESIAN_POINT ( 'NONE',  ( -8.478337820821147730, 185.2758271473933007, 323.2502905065526875 ) ) ;
#15972=CARTESIAN_POINT ( 'NONE',  ( -14.95284176865328263, 180.0521946526295949, 316.6167187968075041 ) ) ;
#15973=CARTESIAN_POINT ( 'NONE',  ( 12.11216763350604175, 187.6476608629002385, 304.8965484581246415 ) ) ;
#16000=CARTESIAN_POINT ( 'NONE',  ( 21.12819794574845389, 168.6979899673408738, 317.6497408708420380 ) ) ;
#16024=CARTESIAN_POINT ( 'NONE',  ( -25.88280235575286170, 324.3728210164380243, 319.3441878704100532 ) ) ;
#16048=CARTESIAN_POINT ( 'NONE',  ( 18.83139044548908814, 185.0137141601130111, 311.0664150449422891 ) ) ;
#16052=CARTESIAN_POINT ( 'NONE',  ( -9.634491729107175217, 187.4432466547973490, 321.1725384739820015 ) ) ;
#16066=DIRECTION ( 'NONE',  ( 0.3101392564284309317, 0.9506461370142480494, -0.009250070373105347826 ) ) ;
#16078=CARTESIAN_POINT ( 'NONE',  ( -15.10364691323318453, 179.7443129775531077, 313.4557914687290463 ) ) ;
#16081=CARTESIAN_POINT ( 'NONE',  ( -3.321556572323998591, 326.9070248174119797, 307.9735416348814852 ) ) ;
#16082=CARTESIAN_POINT ( 'NONE',  ( -15.06363346259513314, 179.7749131191535525, 316.0688698145405056 ) ) ;
#16106=CARTESIAN_POINT ( 'NONE',  ( -0.8458322068501320512, 327.1987054268951169, 310.0943410453546107 ) ) ;
#16118=SPHERICAL_SURFACE ( 'NONE', #14394, 11.00000000000000533 ) ;
#16127=DIRECTION ( 'NONE',  ( 0.3101392564284310982, 0.9506461370142479383, -0.009250070373107712254 ) ) ;
#16131=CARTESIAN_POINT ( 'NONE',  ( -23.19743147896374680, 324.6326046529285350, 307.6196804043323709 ) ) ;
#16145=DIRECTION ( 'NONE',  ( -0.01292394549866745720, -0.005513023399720816918, -0.9999012842304692006 ) ) ;
#16148=AXIS2_PLACEMENT_3D ( 'NONE', #12146, #18915, #16999 ) ;
#16159=CARTESIAN_POINT ( 'NONE',  ( 19.35430270680923925, 183.2211243877775075, 311.5661513781196845 ) ) ;
#16172=EDGE_CURVE ( 'NONE', #3176, #6678, #854, .T. ) ;
#16182=CARTESIAN_POINT ( 'NONE',  ( 11.80593078190077883, 176.3657686503914874, 324.4440941186779810 ) ) ;
#16184=CARTESIAN_POINT ( 'NONE',  ( 12.28794424968258170, 188.3253985970229678, 320.9523548641618049 ) ) ;
#16191=CARTESIAN_POINT ( 'NONE',  ( -9.161099694250802727, 184.8065847297386881, 323.2196502909779952 ) ) ;
#16197=CARTESIAN_POINT ( 'NONE',  ( -12.81093929260451780, 184.2871116315758115, 320.0335541037995313 ) ) ;
#16199=CARTESIAN_POINT ( 'NONE',  ( -14.18925437717659577, 181.7892865527765025, 318.4638477695755796 ) ) ;
#16207=CARTESIAN_POINT ( 'NONE',  ( 11.93555147538424777, 188.0368403985024486, 306.1756385059576360 ) ) ;
#16224=CARTESIAN_POINT ( 'NONE',  ( 3.898201936395599532, 166.6627968962365287, 301.5965304707955852 ) ) ;
#16235=AXIS2_PLACEMENT_3D ( 'NONE', #20326, #3095, #4583 ) ;
#16238=CARTESIAN_POINT ( 'NONE',  ( -5.563703806607757762, 326.7005119474488311, 320.3383740725303710 ) ) ;
#16275=DIRECTION ( 'NONE',  ( -0.3102455404053342525, -0.9506564598521393128, 0.000000000000000000 ) ) ;
#16278=CARTESIAN_POINT ( 'NONE',  ( 18.14697571336121840, 185.8659025024385585, 310.2548099270366606 ) ) ;
#16285=VECTOR ( 'NONE', #6298, 1000.000000000000114 ) ;
#16295=EDGE_CURVE ( 'NONE', #11132, #19478, #7373, .T. ) ;
#16303=DIRECTION ( 'NONE',  ( -0.01292394549866727679, -0.005513023399720743192, -0.9999012842304693116 ) ) ;
#16317=CARTESIAN_POINT ( 'NONE',  ( -15.01362440653151786, 178.7143772909413713, 313.5209786370710958 ) ) ;
#16319=ORIENTED_EDGE ( 'NONE', *, *, #16398, .T. ) ;
#16344=AXIS2_PLACEMENT_3D ( 'NONE', #20405, #11592, #20303 ) ;
#16384=DIRECTION ( 'NONE',  ( -0.9506032891036972909, 0.3102281881984321754, 0.01057629388542893900 ) ) ;
#16387=CARTESIAN_POINT ( 'NONE',  ( 19.76541804458917539, 182.9254338870941297, 318.4526189355386236 ) ) ;
#16398=EDGE_CURVE ( 'NONE', #15431, #13179, #21085, .T. ) ;
#16407=DIRECTION ( 'NONE',  ( -0.9934404589540162256, -0.1135548637187057258, 0.01346653032743021748 ) ) ;
#16410=EDGE_CURVE ( 'NONE', #3703, #4735, #11655, .T. ) ;
#16421=CARTESIAN_POINT ( 'NONE',  ( -13.17740673624774317, 181.2762379934293335, 309.7265655061761436 ) ) ;
#16434=CARTESIAN_POINT ( 'NONE',  ( -14.62480137330870456, 179.3298053622281714, 309.9632843756066904 ) ) ;
#16457=FACE_OUTER_BOUND ( 'NONE', #12145, .T. ) ;
#16468=CARTESIAN_POINT ( 'NONE',  ( -22.66159625276162970, 324.6936785073799001, 307.5691494985305781 ) ) ;
#16492=CARTESIAN_POINT ( 'NONE',  ( 19.91678837892234810, 183.5273396323361794, 313.8466901984123751 ) ) ;
#16498=ORIENTED_EDGE ( 'NONE', *, *, #21689, .T. ) ;
#16499=DIRECTION ( 'NONE',  ( -0.9934404589540163366, -0.1135548637187058507, 0.01346653032743036667 ) ) ;
#16503=LINE ( 'NONE', #13068, #13392 ) ;
#16530=CARTESIAN_POINT ( 'NONE',  ( -10.03417356088257506, 184.3143220770519122, 308.0707497775335355 ) ) ;
#16546=CARTESIAN_POINT ( 'NONE',  ( -14.00607518686419084, 180.2131691732588195, 308.7767599486462586 ) ) ;
#16553=B_SPLINE_CURVE_WITH_KNOTS ( 'NONE', 3,
 ( #19292, #20785, #5041, #12074, #19062, #11930, #1258, #6841, #13863, #4554, #18580, #10087, #8446, #15602, #8246, #4768, #15495, #22446 ),
 .UNSPECIFIED., .F., .F.,
 ( 4, 2, 2, 2, 2, 2, 2, 2, 4 ),
 ( 0.000000000000000000, 0.1250000000000000000, 0.2500000000000000000, 0.3750000000000000000, 0.5000000000000000000, 0.6250000000000000000, 0.7500000000000000000, 0.8750000000000000000, 1.000000000000000000 ),
 .UNSPECIFIED. ) ;
#16555=ORIENTED_EDGE ( 'NONE', *, *, #17533, .F. ) ;
#16563=AXIS2_PLACEMENT_3D ( 'NONE', #15701, #12015, #16985 ) ;
#16573=ORIENTED_EDGE ( 'NONE', *, *, #3343, .T. ) ;
#16574=DIRECTION ( 'NONE',  ( -0.01292394549866727679, -0.005513023399720742325, -0.9999012842304692006 ) ) ;
#16602=AXIS2_PLACEMENT_3D ( 'NONE', #19816, #4086, #20155 ) ;
#16618=CARTESIAN_POINT ( 'NONE',  ( 18.67701816413673654, 183.9365283982369021, 318.2129698699529285 ) ) ;
#16635=FACE_OUTER_BOUND ( 'NONE', #8507, .T. ) ;
#16643=AXIS2_PLACEMENT_3D ( 'NONE', #221, #7217, #17923 ) ;
#16647=CARTESIAN_POINT ( 'NONE',  ( -9.712210512681874519, 187.7615446298876236, 321.1679357793473173 ) ) ;
#16652=CARTESIAN_POINT ( 'NONE',  ( -13.42494546845840020, 180.9759964141439923, 309.9922123620679031 ) ) ;
#16658=DIRECTION ( 'NONE',  ( 0.01292394549866727679, 0.005513023399720742325, 0.9999012842304692006 ) ) ;
#16663=CARTESIAN_POINT ( 'NONE',  ( 12.05007958101849574, 187.6699938018584533, 304.8922276890921239 ) ) ;
#16677=ORIENTED_EDGE ( 'NONE', *, *, #16410, .T. ) ;
#16692=CARTESIAN_POINT ( 'NONE',  ( 13.18210494705709301, 190.2238003902018875, 320.8376354884886723 ) ) ;
#16704=CARTESIAN_POINT ( 'NONE',  ( -8.474913151513398191, 165.2748993292589148, 308.3080180880245962 ) ) ;
#16708=CIRCLE ( 'NONE', #2008, 10.71774939102741264 ) ;
#16726=CARTESIAN_POINT ( 'NONE',  ( 19.87237553197154938, 182.8168944290782179, 318.2233073528176419 ) ) ;
#16759=CARTESIAN_POINT ( 'NONE',  ( -14.07499434214214240, 182.1903141478447310, 310.6856384327238629 ) ) ;
#16775=DIRECTION ( 'NONE',  ( -0.3101392564284313758, -0.9506461370142479383, 0.009250070373107143265 ) ) ;
#16789=FACE_OUTER_BOUND ( 'NONE', #13191, .T. ) ;
#16809=EDGE_LOOP ( 'NONE', ( #10805, #14377, #21929, #20566, #6009 ) ) ;
#16813=ORIENTED_EDGE ( 'NONE', *, *, #17341, .T. ) ;
#16826=CARTESIAN_POINT ( 'NONE',  ( 19.38059109545055492, 183.2942308163235055, 317.1334150972197676 ) ) ;
#16834=CARTESIAN_POINT ( 'NONE',  ( -10.02114103959053182, 187.8727639482237635, 308.1601374225635368 ) ) ;
#16836=CARTESIAN_POINT ( 'NONE',  ( 3.943435745640934798, 166.6820924781355302, 305.0961849656022764 ) ) ;
#16861=CARTESIAN_POINT ( 'NONE',  ( -14.45874313190398297, 179.5722162953435088, 309.6207302340725391 ) ) ;
#16876=CARTESIAN_POINT ( 'NONE',  ( 11.93152547184112322, 187.7152878153667643, 304.8830991845499625 ) ) ;
#16886=CIRCLE ( 'NONE', #10267, 120.0000000000000142 ) ;
#16888=CARTESIAN_POINT ( 'NONE',  ( -9.785137964318257886, 187.5706118828227318, 308.1235300825433683 ) ) ;
#16895=CARTESIAN_POINT ( 'NONE',  ( 15.92090764981139017, 188.3996504711684281, 320.0687762302596866 ) ) ;
#16907=ORIENTED_EDGE ( 'NONE', *, *, #1370, .T. ) ;
#16952=CARTESIAN_POINT ( 'NONE',  ( 3.212657888003040974, 175.3835135662012874, 324.5595797047259907 ) ) ;
#16956=ORIENTED_EDGE ( 'NONE', *, *, #6726, .T. ) ;
#16960=AXIS2_PLACEMENT_3D ( 'NONE', #12994, #21559, #19724 ) ;
#16984=ORIENTED_EDGE ( 'NONE', *, *, #15326, .F. ) ;
#16985=DIRECTION ( 'NONE',  ( 0.3101392564284310982, 0.9506461370142479383, -0.009250070373107712254 ) ) ;
#16986=CARTESIAN_POINT ( 'NONE',  ( -8.409519743373715883, 185.4801247956302745, 308.0432246570530310 ) ) ;
#16999=DIRECTION ( 'NONE',  ( 0.9506868100732489557, -0.3101525256269085928, 0.000000000000000000 ) ) ;
#17012=CARTESIAN_POINT ( 'NONE',  ( -25.54600055714195506, 324.4124461427009010, 319.6189258610973525 ) ) ;
#17021=CARTESIAN_POINT ( 'NONE',  ( 14.55162269530302943, 189.3886954157946434, 320.5815939255251124 ) ) ;
#17027=DIRECTION ( 'NONE',  ( -0.3102455404053335308, -0.9506564598521395348, 0.000000000000000000 ) ) ;
#17055=VERTEX_POINT ( 'NONE', #20860 ) ;
#17067=VERTEX_POINT ( 'NONE', #4662 ) ;
#17068=AXIS2_PLACEMENT_3D ( 'NONE', #2880, #6104, #13131 ) ;
#17082=CARTESIAN_POINT ( 'NONE',  ( -13.36217923100928928, 326.0172268059896510, 372.0162718331554288 ) ) ;
#17091=CARTESIAN_POINT ( 'NONE',  ( -8.468920434824459775, 185.4410853633842464, 308.0359439383103108 ) ) ;
#17097=CARTESIAN_POINT ( 'NONE',  ( 15.07021670940958913, 186.4546686254222720, 322.6590458595396740 ) ) ;
#17102=CARTESIAN_POINT ( 'NONE',  ( 14.16699832106635526, 189.6353986260119484, 320.6813409114420210 ) ) ;
#17114=ADVANCED_FACE ( 'NONE', ( #5349 ), #14569, .F. ) ;
#17190=VERTEX_POINT ( 'NONE', #18125 ) ;
#17196=CARTESIAN_POINT ( 'NONE',  ( 15.34006562386835881, 188.8538180965162780, 320.3317479991936239 ) ) ;
#17240=ADVANCED_FACE ( 'NONE', ( #20357 ), #11836, .T. ) ;
#17243=LINE ( 'NONE', #8608, #9748 ) ;
#17247=CIRCLE ( 'NONE', #18354, 1.999999999999998224 ) ;
#17257=CARTESIAN_POINT ( 'NONE',  ( -9.955606456259319614, 184.2243514862264533, 323.1466302186144617 ) ) ;
#17266=CIRCLE ( 'NONE', #6240, 10.00000000000001421 ) ;
#17268=EDGE_LOOP ( 'NONE', ( #17549, #15465, #18252, #11896 ) ) ;
#17271=CARTESIAN_POINT ( 'NONE',  ( 17.00040199784601214, 187.3380220790077431, 319.4296498798100288 ) ) ;
#17292=B_SPLINE_CURVE_WITH_KNOTS ( 'NONE', 3,
 ( #22308, #22089, #15474, #1109 ),
 .UNSPECIFIED., .F., .F.,
 ( 4, 4 ),
 ( 0.000000000000000000, 0.0001181342984831720616 ),
 .UNSPECIFIED. ) ;
#17300=CARTESIAN_POINT ( 'NONE',  ( 11.72327481064200683, 187.7930371575377535, 304.8675929460329144 ) ) ;
#17318=B_SPLINE_CURVE_WITH_KNOTS ( 'NONE', 3,
 ( #328, #7319, #908, #7444, #21770, #16207, #4213, #7658, #19708, #3977, #9154, #11241, #11001, #674, #14936, #9633, #7898, #5942 ),
 .UNSPECIFIED., .F., .F.,
 ( 4, 2, 2, 2, 2, 2, 2, 2, 4 ),
 ( -3.889482208294626299E-05, 0.0005389813427436562733, 0.001116857507570258789, 0.001694733672396861197, 0.002272609837223463821, 0.002850486002050066445, 0.003428362166876668636, 0.004006238331703271260, 0.004584114496529873885 ),
 .UNSPECIFIED. ) ;
#17320=PLANE ( 'NONE',  #4715 ) ;
#17337=CARTESIAN_POINT ( 'NONE',  ( 20.60016704620528571, 181.9681718854236294, 313.0792466296721841 ) ) ;
#17341=EDGE_CURVE ( 'NONE', #17190, #18283, #15779, .T. ) ;
#17349=DIRECTION ( 'NONE',  ( -0.01292394549866727679, -0.005513023399720743192, -0.9999012842304693116 ) ) ;
#17381=CARTESIAN_POINT ( 'NONE',  ( -8.663423201070779456, 185.1548080327998207, 323.2462545196998462 ) ) ;
#17385=FACE_OUTER_BOUND ( 'NONE', #14354, .T. ) ;
#17393=CARTESIAN_POINT ( 'NONE',  ( 17.14877061339265651, 185.1529327208830580, 321.7930803067964689 ) ) ;
#17417=VERTEX_POINT ( 'NONE', #12090 ) ;
#17419=FACE_OUTER_BOUND ( 'NONE', #295, .T. ) ;
#17430=ORIENTED_EDGE ( 'NONE', *, *, #5007, .T. ) ;
#17439=CARTESIAN_POINT ( 'NONE',  ( 16.39634482804417104, 187.9401017119211019, 319.7988598509799090 ) ) ;
#17444=ADVANCED_FACE ( 'NONE', ( #18995 ), #6231, .T. ) ;
#17456=ORIENTED_EDGE ( 'NONE', *, *, #18206, .F. ) ;
#17457=CARTESIAN_POINT ( 'NONE',  ( 20.32642875375586655, 182.3364184945779698, 317.0345009060944221 ) ) ;
#17479=CARTESIAN_POINT ( 'NONE',  ( -13.92525281995234820, 325.7770340667113942, 328.4523304068723064 ) ) ;
#17483=CARTESIAN_POINT ( 'NONE',  ( -0.5919341415252730165, 327.2293163420105770, 310.4847058774875563 ) ) ;
#17494=DIRECTION ( 'NONE',  ( 0.3101392564284310982, 0.9506461370142479383, -0.009250070373107712254 ) ) ;
#17502=CARTESIAN_POINT ( 'NONE',  ( -7.771066633828587200, 165.4076424879065996, 321.2562038772189226 ) ) ;
#17506=ORIENTED_EDGE ( 'NONE', *, *, #14081, .T. ) ;
#17513=EDGE_LOOP ( 'NONE', ( #4521, #5176, #18811, #8796 ) ) ;
#17517=CARTESIAN_POINT ( 'NONE',  ( 17.86990006708586165, 186.2024540464122708, 309.9547898294551942 ) ) ;
#17518=VERTEX_POINT ( 'NONE', #13628 ) ;
#17527=CARTESIAN_POINT ( 'NONE',  ( 13.57515324494882769, 187.0243046317364701, 305.1469784402785308 ) ) ;
#17529=MANIFOLD_SOLID_BREP ( 'Stock-MAS-425-1', #6212 ) ;
#17533=EDGE_CURVE ( 'NONE', #5229, #4135, #17782, .T. ) ;
#17549=ORIENTED_EDGE ( 'NONE', *, *, #17947, .T. ) ;
#17556=DIRECTION ( 'NONE',  ( -0.01292394549866745720, -0.005513023399720816918, -0.9999012842304692006 ) ) ;
#17562=CARTESIAN_POINT ( 'NONE',  ( -5.817627660042380633, 326.6189945014031082, 307.3338991736922594 ) ) ;
#17563=CARTESIAN_POINT ( 'NONE',  ( -15.23311339992631197, 178.2575602159987227, 317.4829393096611625 ) ) ;
#17566=CARTESIAN_POINT ( 'NONE',  ( 13.80207227627342803, 186.9166813556422255, 305.2099784584296458 ) ) ;
#17577=DIRECTION ( 'NONE',  ( -0.9934404589540162256, -0.1135548637187057258, 0.01346653032743021748 ) ) ;
#17594=CARTESIAN_POINT ( 'NONE',  ( 17.20172502694573780, 168.2615119090760345, 320.7598891025185708 ) ) ;
#17615=CARTESIAN_POINT ( 'NONE',  ( -11.16028402830248289, 165.0151156927683473, 320.0325255541022784 ) ) ;
#17628=CARTESIAN_POINT ( 'NONE',  ( 19.80886166575337981, 183.6751623284734194, 313.1938135270697785 ) ) ;
#17629=EDGE_CURVE ( 'NONE', #9497, #3176, #20463, .T. ) ;
#17640=CARTESIAN_POINT ( 'NONE',  ( 13.39998349785021681, 190.1428121419461093, 307.9026663383229447 ) ) ;
#17653=CARTESIAN_POINT ( 'NONE',  ( -9.157834647979710141, 186.7064098873641456, 321.4482401296887701 ) ) ;
#17667=EDGE_CURVE ( 'NONE', #18283, #126, #19783, .T. ) ;
#17672=CARTESIAN_POINT ( 'NONE',  ( 12.31279916714637146, 188.3155709156417856, 320.9502181276351962 ) ) ;
#17679=CARTESIAN_POINT ( 'NONE',  ( -8.521464884669340378, 185.2469399555467646, 323.2491637953797863 ) ) ;
#17682=VERTEX_POINT ( 'NONE', #7516 ) ;
#17683=CARTESIAN_POINT ( 'NONE',  ( -10.63979810906646328, 187.2538219846114487, 308.2525677622306830 ) ) ;
#17689=CARTESIAN_POINT ( 'NONE',  ( -15.31456691273178450, 178.2055753609038220, 312.1839202388429726 ) ) ;
#17690=AXIS2_PLACEMENT_3D ( 'NONE', #20799, #22278, #8508 ) ;
#17692=CIRCLE ( 'NONE', #809, 22.49999999999999645 ) ;
#17719=CARTESIAN_POINT ( 'NONE',  ( 20.34336355497194049, 168.6127106875439381, 318.7583842999745229 ) ) ;
#17723=CIRCLE ( 'NONE', #7797, 25.50000000000000000 ) ;
#17725=ORIENTED_EDGE ( 'NONE', *, *, #14168, .F. ) ;
#17743=CARTESIAN_POINT ( 'NONE',  ( -11.79244185255453203, 164.9406916783147494, 319.5044911414121884 ) ) ;
#17769=CARTESIAN_POINT ( 'NONE',  ( 19.08844512645451275, 183.3985617639965540, 309.1678998821465711 ) ) ;
#17782=B_SPLINE_CURVE_WITH_KNOTS ( 'NONE', 3,
 ( #19453, #7173, #1893, #52, #10739, #20828, #9107 ),
 .UNSPECIFIED., .F., .F.,
 ( 4, 3, 4 ),
 ( 0.000000000000000000, 2.978207829266235889E-05, 2.984123798783903494E-05 ),
 .UNSPECIFIED. ) ;
#17805=CARTESIAN_POINT ( 'NONE',  ( -13.88059897197513060, 182.5799557881418593, 310.4051692506089921 ) ) ;
#17810=CARTESIAN_POINT ( 'NONE',  ( -14.96620062107659876, 178.7509044520041357, 316.1111495142839658 ) ) ;
#17812=CARTESIAN_POINT ( 'NONE',  ( 20.64603878514330404, 181.9656304078110338, 315.4952833946043143 ) ) ;
#17822=VERTEX_POINT ( 'NONE', #1206 ) ;
#17823=DIRECTION ( 'NONE',  ( 0.9506032891036972909, -0.3102281881984320644, -0.01057629388542894074 ) ) ;
#17859=CARTESIAN_POINT ( 'NONE',  ( -10.83342074598470184, 165.0533908189748900, 320.2543728156808243 ) ) ;
#17883=CARTESIAN_POINT ( 'NONE',  ( 12.31508922632070302, 187.5663303611497383, 304.9177876444722983 ) ) ;
#17892=B_SPLINE_CURVE_WITH_KNOTS ( 'NONE', 3,
 ( #20189, #6434, #13444, #1378, #20412, #4671, #11704, #18699, #2969, #9985, #13547, #8352, #20527, #4459, #17012, #8261, #20653, #11832 ),
 .UNSPECIFIED., .F., .F.,
 ( 4, 2, 2, 2, 2, 2, 2, 2, 4 ),
 ( 0.000000000000000000, 0.1250000000000000000, 0.2500000000000000000, 0.3750000000000000000, 0.5000000000000000000, 0.6250000000000000000, 0.7500000000000000000, 0.8750000000000000000, 1.000000000000000000 ),
 .UNSPECIFIED. ) ;
#17899=DIRECTION ( 'NONE',  ( -0.01292394549866745720, -0.005513023399720816918, -0.9999012842304692006 ) ) ;
#17914=CARTESIAN_POINT ( 'NONE',  ( -14.48496598153953485, 181.1498399189628969, 317.9007409887333893 ) ) ;
#17916=DIRECTION ( 'NONE',  ( -0.01292394549866754394, -0.005513023399720772683, -0.9999012842304692006 ) ) ;
#17923=DIRECTION ( 'NONE',  ( 0.3102455404053300891, 0.9506564598521406451, 0.000000000000000000 ) ) ;
#17933=DIRECTION ( 'NONE',  ( 0.9934404589540162256, 0.1135548637187060589, -0.01346653032743021922 ) ) ;
#17939=ORIENTED_EDGE ( 'NONE', *, *, #22361, .T. ) ;
#17947=EDGE_CURVE ( 'NONE', #5612, #7136, #15314, .T. ) ;
#17961=CARTESIAN_POINT ( 'NONE',  ( -13.55891735653775676, 164.7118933236453415, 312.8669722336247219 ) ) ;
#17975=CIRCLE ( 'NONE', #16148, 10.99999999999999822 ) ;
#17987=CARTESIAN_POINT ( 'NONE',  ( 14.87756490533177356, 186.3606781135739823, 305.6069114145042818 ) ) ;
#18008=LINE ( 'NONE', #16182, #2700 ) ;
#18023=CARTESIAN_POINT ( 'NONE',  ( -15.53263949983598202, 177.8010796364676480, 313.8283261121160876 ) ) ;
#18049=AXIS2_PLACEMENT_3D ( 'NONE', #10314, #92, #19028 ) ;
#18052=ORIENTED_EDGE ( 'NONE', *, *, #5168, .T. ) ;
#18057=( GEOMETRIC_REPRESENTATION_CONTEXT ( 3 ) GLOBAL_UNCERTAINTY_ASSIGNED_CONTEXT ( ( #6316 ) ) GLOBAL_UNIT_ASSIGNED_CONTEXT ( ( #10965, #11422, #6025 ) ) REPRESENTATION_CONTEXT ( 'NONE', 'WORKASPACE' ) );
#18059=AXIS2_PLACEMENT_3D ( 'NONE', #20537, #4680, #1164 ) ;
#18070=EDGE_CURVE ( 'NONE', #22032, #13714, #2644, .T. ) ;
#18086=CARTESIAN_POINT ( 'NONE',  ( 12.81503532323078964, 190.4972571607467842, 307.8483445055002221 ) ) ;
#18105=CARTESIAN_POINT ( 'NONE',  ( 20.02685672050394317, 182.6349384657623887, 315.1934792567789714 ) ) ;
#18110=AXIS2_PLACEMENT_3D ( 'NONE', #12055, #14012, #6984 ) ;
#18125=CARTESIAN_POINT ( 'NONE',  ( -22.60047370202423167, 329.4438419316639965, 414.4311550204333798 ) ) ;
#18140=CARTESIAN_POINT ( 'NONE',  ( -11.48960883379135467, 186.2785219672419146, 308.5185337839570252 ) ) ;
#18143=CARTESIAN_POINT ( 'NONE',  ( -11.07366896422823288, 186.7668193309826279, 308.3749965093444416 ) ) ;
#18152=CARTESIAN_POINT ( 'NONE',  ( -4.397807287087292849, 165.8073468632632910, 324.7107454954286823 ) ) ;
#18171=SHAPE_DEFINITION_REPRESENTATION ( #21615, #15037 ) ;
#18198=ORIENTED_EDGE ( 'NONE', *, *, #6838, .F. ) ;
#18203=VERTEX_POINT ( 'NONE', #15647 ) ;
#18206=EDGE_CURVE ( 'NONE', #8155, #9852, #5377, .T. ) ;
#18213=CARTESIAN_POINT ( 'NONE',  ( 19.86028698246260404, 182.7578626415639178, 312.8315258640758429 ) ) ;
#18218=CARTESIAN_POINT ( 'NONE',  ( -9.995692194476635706, 187.8898849410517471, 308.1575541326492953 ) ) ;
#18241=CARTESIAN_POINT ( 'NONE',  ( -15.14040723921782572, 178.5077077566731418, 311.4171169843866664 ) ) ;
#18245=ADVANCED_FACE ( 'NONE', ( #4230 ), #1548, .T. ) ;
#18252=ORIENTED_EDGE ( 'NONE', *, *, #14431, .F. ) ;
#18254=CARTESIAN_POINT ( 'NONE',  ( -12.64949829888728772, 181.7347035077120267, 322.1854682947845845 ) ) ;
#18283=VERTEX_POINT ( 'NONE', #4112 ) ;
#18302=CARTESIAN_POINT ( 'NONE',  ( -18.18280553459775106, 164.2235859539597413, 322.8974543720026418 ) ) ;
#18306=CARTESIAN_POINT ( 'NONE',  ( -9.995692194476635706, 187.8898849410517471, 308.1575541326492953 ) ) ;
#18308=CARTESIAN_POINT ( 'NONE',  ( 19.16750076320854035, 183.4954371053536875, 317.5119934807448772 ) ) ;
#18322=EDGE_CURVE ( 'NONE', #1264, #22032, #21678, .T. ) ;
#18340=CARTESIAN_POINT ( 'NONE',  ( -14.99641971449742783, 178.7475833985533029, 310.9402587844948584 ) ) ;
#18341=ORIENTED_EDGE ( 'NONE', *, *, #8979, .T. ) ;
#18347=VECTOR ( 'NONE', #18725, 1000.000000000000114 ) ;
#18354=AXIS2_PLACEMENT_3D ( 'NONE', #209, #10885, #556 ) ;
#18360=ADVANCED_FACE ( 'NONE', ( #18485 ), #2749, .F. ) ;
#18361=CARTESIAN_POINT ( 'NONE',  ( -15.23197394876478761, 178.3512841404416349, 311.7746290397823259 ) ) ;
#18387=CARTESIAN_POINT ( 'NONE',  ( 4.195452682864946325, 166.7895964344300808, 324.5942600080963985 ) ) ;
#18402=CARTESIAN_POINT ( 'NONE',  ( -22.53299579847311307, 324.7083362324482323, 307.5570220811381432 ) ) ;
#18412=VECTOR ( 'NONE', #17349, 999.9999999999998863 ) ;
#18431=CARTESIAN_POINT ( 'NONE',  ( 20.16092468778748170, 182.5150849490638620, 317.5062687794200542 ) ) ;
#18454=LINE ( 'NONE', #21860, #11347 ) ;
#18466=CARTESIAN_POINT ( 'NONE',  ( -13.42770478899201514, 180.9551723136957264, 307.9573190744438875 ) ) ;
#18475=AXIS2_PLACEMENT_3D ( 'NONE', #12404, #14137, #12177 ) ;
#18479=CARTESIAN_POINT ( 'NONE',  ( 12.78096684794300941, 190.5101800092401731, 307.8461504866875202 ) ) ;
#18481=CARTESIAN_POINT ( 'NONE',  ( -8.523216527044569446, 185.4125284852929099, 305.1540476800932424 ) ) ;
#18485=FACE_OUTER_BOUND ( 'NONE', #16809, .T. ) ;
#18488=AXIS2_PLACEMENT_3D ( 'NONE', #19921, #4296, #9368 ) ;
#18492=ADVANCED_FACE ( 'NONE', ( #16635 ), #15513, .T. ) ;
#18501=VECTOR ( 'NONE', #22054, 1000.000000000000227 ) ;
#18544=CARTESIAN_POINT ( 'NONE',  ( 13.77150744767909352, 159.1779288738256923, 324.5124548241344655 ) ) ;
#18545=CARTESIAN_POINT ( 'NONE',  ( 20.49956196390964891, 182.0660229792639768, 312.5168992756803732 ) ) ;
#18548=ORIENTED_EDGE ( 'NONE', *, *, #3608, .T. ) ;
#18573=CARTESIAN_POINT ( 'NONE',  ( -13.02319649578260119, 181.4398012765341832, 307.4785573789200157 ) ) ;
#18576=ORIENTED_EDGE ( 'NONE', *, *, #19142, .T. ) ;
#18578=CARTESIAN_POINT ( 'NONE',  ( 13.64212105858742241, 187.1241579171488070, 322.8665338120699744 ) ) ;
#18580=CARTESIAN_POINT ( 'NONE',  ( 0.1403038029401039999, 327.3197362253691836, 312.1404394970679164 ) ) ;
#18584=CARTESIAN_POINT ( 'NONE',  ( 12.62937233005813908, 190.5670816176184132, 307.8363845662464087 ) ) ;
#18585=CARTESIAN_POINT ( 'NONE',  ( -15.51253772856980362, 177.8410551567861830, 313.5641263009300701 ) ) ;
#18594=CARTESIAN_POINT ( 'NONE',  ( -9.483901319675773323, 187.1048918696979229, 307.9736811914152668 ) ) ;
#18608=ORIENTED_EDGE ( 'NONE', *, *, #11747, .F. ) ;
#18639=EDGE_LOOP ( 'NONE', ( #17506, #6483, #17939, #19831, #14500, #8640, #18548, #18052, #17456, #7816 ) ) ;
#18663=ORIENTED_EDGE ( 'NONE', *, *, #15237, .F. ) ;
#18673=CARTESIAN_POINT ( 'NONE',  ( -8.248824808275418974, 185.5853417291986887, 308.0251062239191810 ) ) ;
#18679=CARTESIAN_POINT ( 'NONE',  ( 15.75623612227090575, 186.0822479155119140, 322.5113043239726380 ) ) ;
#18686=CARTESIAN_POINT ( 'NONE',  ( -14.80339701313337386, 179.0542959306228568, 310.3963275995649838 ) ) ;
#18699=CARTESIAN_POINT ( 'NONE',  ( -28.40747727069632589, 324.0565921083061198, 312.5274174544723564 ) ) ;
#18715=AXIS2_PLACEMENT_3D ( 'NONE', #3402, #1691, #19246 ) ;
#18725=DIRECTION ( 'NONE',  ( 0.1136178953597579422, -0.9935164314186355483, 0.004009283626633659663 ) ) ;
#18739=VERTEX_POINT ( 'NONE', #8880 ) ;
#18741=CARTESIAN_POINT ( 'NONE',  ( -8.991637549221998427, 184.9283712355567104, 323.2327844428430126 ) ) ;
#18797=CARTESIAN_POINT ( 'NONE',  ( -8.380575353881514644, 185.4992511567469080, 308.0384472719858309 ) ) ;
#18811=ORIENTED_EDGE ( 'NONE', *, *, #13175, .F. ) ;
#18832=CARTESIAN_POINT ( 'NONE',  ( 13.11455560745687876, 190.2624259001582345, 320.8439992888508527 ) ) ;
#18833=FACE_OUTER_BOUND ( 'NONE', #19999, .T. ) ;
#18852=AXIS2_PLACEMENT_3D ( 'NONE', #8615, #1632, #8717 ) ;
#18865=ORIENTED_EDGE ( 'NONE', *, *, #18070, .T. ) ;
#18897=ADVANCED_FACE ( 'NONE', ( #8830 ), #12572, .T. ) ;
#18915=DIRECTION ( 'NONE',  ( -0.3101392564284312647, -0.9506461370142480494, 0.009250070373107143265 ) ) ;
#18919=CIRCLE ( 'NONE', #4974, 20.50000000000000355 ) ;
#18926=CARTESIAN_POINT ( 'NONE',  ( -12.01334469841415498, 182.4622809814591449, 320.5389699414921552 ) ) ;
#18930=EDGE_CURVE ( 'NONE', #1264, #5811, #22093, .T. ) ;
#18942=VERTEX_POINT ( 'NONE', #5364 ) ;
#18995=FACE_OUTER_BOUND ( 'NONE', #11739, .T. ) ;
#19018=CARTESIAN_POINT ( 'NONE',  ( 12.53310868402590827, 188.2157523762948870, 320.9566087149508462 ) ) ;
#19028=DIRECTION ( 'NONE',  ( -0.1136178953597579422, 0.9935164314186355483, -0.004009283626633659663 ) ) ;
#19031=DIRECTION ( 'NONE',  ( 0.3101392564284308762, 0.9506461370142480494, -0.009250070373106863975 ) ) ;
#19042=VERTEX_POINT ( 'NONE', #330 ) ;
#19062=CARTESIAN_POINT ( 'NONE',  ( -1.886058359258391270, 327.1149038793577120, 318.8066435240484111 ) ) ;
#19065=CARTESIAN_POINT ( 'NONE',  ( 21.94165880485012110, 168.7756884006963389, 313.8512965718784926 ) ) ;
#19066=AXIS2_PLACEMENT_3D ( 'NONE', #1374, #8348, #3292 ) ;
#19076=CARTESIAN_POINT ( 'NONE',  ( -9.638276707334691551, 184.4631002042323757, 323.1821100297731846 ) ) ;
#19114=FACE_OUTER_BOUND ( 'NONE', #14376, .T. ) ;
#19125=AXIS2_PLACEMENT_3D ( 'NONE', #18387, #2766, #13017 ) ;
#19130=CARTESIAN_POINT ( 'NONE',  ( -13.98112707844397562, 325.7531995422979207, 324.1294444254230598 ) ) ;
#19142=EDGE_CURVE ( 'NONE', #4735, #6191, #13200, .T. ) ;
#19148=CARTESIAN_POINT ( 'NONE',  ( 16.76385840201456290, 185.2028283229317651, 306.7113249663256056 ) ) ;
#19182=CARTESIAN_POINT ( 'NONE',  ( 21.46898066623532841, 168.7138791228462367, 311.9297967271122047 ) ) ;
#19207=CARTESIAN_POINT ( 'NONE',  ( -13.77044500111245107, 164.6916052361225979, 313.8339224003136678 ) ) ;
#19231=CARTESIAN_POINT ( 'NONE',  ( 11.77922689329016848, 187.8031667290258042, 307.7652408209249870 ) ) ;
#19246=DIRECTION ( 'NONE',  ( 0.3101392564284308762, 0.9506461370142480494, -0.009250070373106863975 ) ) ;
#19255=CARTESIAN_POINT ( 'NONE',  ( 12.94357278854792170, 190.3382146902982583, 320.8588152455632780 ) ) ;
#19259=CARTESIAN_POINT ( 'NONE',  ( -12.58664483627157260, 184.6272112293439704, 320.1917372557448402 ) ) ;
#19260=CARTESIAN_POINT ( 'NONE',  ( 4.169604791867612015, 166.7785703876306513, 322.5944574396354483 ) ) ;
#19265=FACE_OUTER_BOUND ( 'NONE', #18639, .T. ) ;
#19268=CARTESIAN_POINT ( 'NONE',  ( 18.18475692997101589, 184.3587657017563117, 320.8069875086114848 ) ) ;
#19285=ORIENTED_EDGE ( 'NONE', *, *, #8353, .F. ) ;
#19289=FACE_OUTER_BOUND ( 'NONE', #5131, .T. ) ;
#19292=CARTESIAN_POINT ( 'NONE',  ( -5.563703806607757762, 326.7005119474488311, 320.3383740725303710 ) ) ;
#19296=CARTESIAN_POINT ( 'NONE',  ( -3.170773005268938238, 326.9713452165928516, 319.6393817883191559 ) ) ;
#19319=CARTESIAN_POINT ( 'NONE',  ( -24.90374348704198226, 324.4871656374173199, 319.9339819361791228 ) ) ;
#19322=DIRECTION ( 'NONE',  ( -0.01292394549866745720, -0.005513023399720816918, -0.9999012842304692006 ) ) ;
#19324=ADVANCED_FACE ( 'NONE', ( #13763 ), #1578, .T. ) ;
#19345=CARTESIAN_POINT ( 'NONE',  ( 18.36248364585371817, 184.0714940213935904, 310.1538024246328860 ) ) ;
#19363=CARTESIAN_POINT ( 'NONE',  ( 13.09069504930537597, 190.2760544069976163, 320.8462072796203302 ) ) ;
#19372=CARTESIAN_POINT ( 'NONE',  ( -11.21443378733192020, 186.6088958083097680, 308.4147112809631039 ) ) ;
#19375=CARTESIAN_POINT ( 'NONE',  ( 15.77462424665207763, 168.0465177001844665, 307.9256531486020094 ) ) ;
#19376=CARTESIAN_POINT ( 'NONE',  ( -15.03921139472108415, 178.6409456330145531, 315.6521442976429057 ) ) ;
#19399=ORIENTED_EDGE ( 'NONE', *, *, #22511, .F. ) ;
#19412=EDGE_CURVE ( 'NONE', #3703, #7715, #18008, .T. ) ;
#19414=FACE_OUTER_BOUND ( 'NONE', #17513, .T. ) ;
#19429=CARTESIAN_POINT ( 'NONE',  ( -25.69698422022063866, 324.3509299035710001, 308.6536381847947155 ) ) ;
#19444=PRODUCT_DEFINITION_FORMATION_WITH_SPECIFIED_SOURCE ( 'ANY', '', #20165, .NOT_KNOWN. ) ;
#19453=CARTESIAN_POINT ( 'NONE',  ( 13.01890817498768449, 190.3110758050131892, 320.8522954438618058 ) ) ;
#19455=CARTESIAN_POINT ( 'NONE',  ( 13.46034337553667193, 187.1166012126664668, 307.7207322155608153 ) ) ;
#19478=VERTEX_POINT ( 'NONE', #6042 ) ;
#19480=DIRECTION ( 'NONE',  ( -0.9934404589540162256, -0.1135548637187057258, 0.01346653032743021748 ) ) ;
#19481=CARTESIAN_POINT ( 'NONE',  ( -11.40735840365825915, 183.0524750669056004, 320.8439791889416028 ) ) ;
#19486=CARTESIAN_POINT ( 'NONE',  ( -14.04492576652437918, 182.2513542422996693, 310.6408630182388038 ) ) ;
#19490=CARTESIAN_POINT ( 'NONE',  ( 17.98832021580386353, 168.3016772219343693, 308.4219264720497904 ) ) ;
#19491=CARTESIAN_POINT ( 'NONE',  ( -15.09479064048255381, 179.6969842254679861, 315.8799336093683792 ) ) ;
#19508=AXIS2_PLACEMENT_3D ( 'NONE', #12887, #16574, #5977 ) ;
#19526=CARTESIAN_POINT ( 'NONE',  ( 16.60733960726993530, 168.1940330716068388, 320.8824762435588127 ) ) ;
#19549=CARTESIAN_POINT ( 'NONE',  ( -10.33200872664665049, 165.0651399145666005, 308.9564794664337342 ) ) ;
#19550=VERTEX_POINT ( 'NONE', #6270 ) ;
#19558=ORIENTED_EDGE ( 'NONE', *, *, #5020, .F. ) ;
#19566=DIRECTION ( 'NONE',  ( 0.3101392564284308762, 0.9506461370142480494, -0.009250070373106863975 ) ) ;
#19569=CARTESIAN_POINT ( 'NONE',  ( 19.13497996244607080, 183.4159916094967571, 311.1842790287917069 ) ) ;
#19587=EDGE_CURVE ( 'NONE', #6191, #7136, #7636, .T. ) ;
#19592=DIRECTION ( 'NONE',  ( 0.09199399308265900077, -0.9957502728239346901, 0.004301093787334665970 ) ) ;
#19599=CARTESIAN_POINT ( 'NONE',  ( -15.03272297201332819, 179.8527073090512545, 316.2340475952451584 ) ) ;
#19603=CARTESIAN_POINT ( 'NONE',  ( -15.17825613376442284, 179.5172115246878377, 314.3122088330735551 ) ) ;
#19619=FACE_OUTER_BOUND ( 'NONE', #5691, .T. ) ;
#19650=CARTESIAN_POINT ( 'NONE',  ( -22.36471611834589623, 324.7801200243509925, 320.5765034992891742 ) ) ;
#19663=CARTESIAN_POINT ( 'NONE',  ( -3.738111129692070822, 157.0756041464990744, 299.7478936930373266 ) ) ;
#19670=CARTESIAN_POINT ( 'NONE',  ( 18.51945795647842274, 183.8831096202368087, 308.3970819915673474 ) ) ;
#19675=CARTESIAN_POINT ( 'NONE',  ( -8.375467013762508017, 185.4549566013130857, 322.9624185535398055 ) ) ;
#19685=DIRECTION ( 'NONE',  ( 0.9934404589540162256, 0.1135548637187060589, -0.01346653032743021922 ) ) ;
#19689=CARTESIAN_POINT ( 'NONE',  ( 12.25812685601325214, 187.6818734834393467, 322.9715098129762509 ) ) ;
#19701=CARTESIAN_POINT ( 'NONE',  ( -15.52316384508689495, 177.7875914134558002, 315.5629757591011639 ) ) ;
#19708=CARTESIAN_POINT ( 'NONE',  ( 12.06934323283736532, 188.4384883516733566, 306.8148419804898026 ) ) ;
#19724=DIRECTION ( 'NONE',  ( 0.3102455404053333088, 0.9506564598521396459, 0.000000000000000000 ) ) ;
#19766=CARTESIAN_POINT ( 'NONE',  ( 12.84378735233264379, 190.4863133572641232, 307.8501959441126701 ) ) ;
#19779=CARTESIAN_POINT ( 'NONE',  ( 13.08424151692359061, 187.2836837763990161, 307.6956580856131040 ) ) ;
#19783=CIRCLE ( 'NONE', #3664, 120.0000000000000142 ) ;
#19816=CARTESIAN_POINT ( 'NONE',  ( -13.89421726780587996, 325.7902730365928505, 330.8534925327304563 ) ) ;
#19818=CARTESIAN_POINT ( 'NONE',  ( -13.66360798539897381, 182.8253664500271043, 319.2043023236377621 ) ) ;
#19831=ORIENTED_EDGE ( 'NONE', *, *, #17533, .T. ) ;
#19836=CARTESIAN_POINT ( 'NONE',  ( -4.880720251855715119, 321.6948272370410109, 320.3571455402721426 ) ) ;
#19840=TOROIDAL_SURFACE ( 'NONE', #17690, 10.00000000000000178, 2.272904689641331188 ) ;
#19862=DIRECTION ( 'NONE',  ( -0.9506032891036972909, 0.3102281881984321754, 0.01057629388542893900 ) ) ;
#19877=EDGE_CURVE ( 'NONE', #5811, #5010, #15567, .T. ) ;
#19896=DIRECTION ( 'NONE',  ( 0.3101392564284313758, 0.9506461370142480494, -0.009250070373107145000 ) ) ;
#19902=CARTESIAN_POINT ( 'NONE',  ( 19.71973137965292366, 182.8876731017876978, 312.3882680660079814 ) ) ;
#19909=CARTESIAN_POINT ( 'NONE',  ( 24.26373134495293726, 168.9906716024700017, 301.3204665990833178 ) ) ;
#19921=CARTESIAN_POINT ( 'NONE',  ( -12.81536461602102683, 326.2504838843369726, 414.3222871145668478 ) ) ;
#19930=CARTESIAN_POINT ( 'NONE',  ( -9.687524877350609742, 187.7773076241416277, 321.1696142754236121 ) ) ;
#19938=CARTESIAN_POINT ( 'NONE',  ( -9.427729116192457681, 184.7790183205190431, 305.3034345195356991 ) ) ;
#19956=CARTESIAN_POINT ( 'NONE',  ( -15.10609485879404801, 178.5662836768142654, 311.3009205210422010 ) ) ;
#19999=EDGE_LOOP ( 'NONE', ( #1503, #15325, #16573, #10195 ) ) ;
#20005=VERTEX_POINT ( 'NONE', #1077 ) ;
#20013=CARTESIAN_POINT ( 'NONE',  ( -10.02941182916328167, 187.9619130446263000, 308.1597555601239833 ) ) ;
#20014=CIRCLE ( 'NONE', #10133, 7.000000000000021316 ) ;
#20016=CARTESIAN_POINT ( 'NONE',  ( 19.77978298930075240, 183.7162053505926735, 313.0775227943956338 ) ) ;
#20048=CARTESIAN_POINT ( 'NONE',  ( -8.597624943140569798, 185.9633400538521641, 321.2390708565524733 ) ) ;
#20054=CARTESIAN_POINT ( 'NONE',  ( -14.30933683530841627, 181.6919563439129490, 311.0896036802490698 ) ) ;
#20093=ORIENTED_EDGE ( 'NONE', *, *, #9823, .F. ) ;
#20115=ORIENTED_EDGE ( 'NONE', *, *, #6988, .T. ) ;
#20118=CARTESIAN_POINT ( 'NONE',  ( 18.31812028490978861, 185.8289673428165543, 318.2867877985925134 ) ) ;
#20128=DIRECTION ( 'NONE',  ( -0.01292394549866742424, -0.005513023399720750999, -0.9999012842304693116 ) ) ;
#20129=CIRCLE ( 'NONE', #8395, 11.78759343285143224 ) ;
#20132=CARTESIAN_POINT ( 'NONE',  ( -9.837386872088778489, 187.7736565290674662, 321.1595949917730763 ) ) ;
#20152=CARTESIAN_POINT ( 'NONE',  ( -8.553411222537889103, 185.9935125942876084, 321.2420807565750351 ) ) ;
#20155=DIRECTION ( 'NONE',  ( 0.3101392564284315978, 0.9506461370142478273, -0.009250070373106959384 ) ) ;
#20161=CARTESIAN_POINT ( 'NONE',  ( -8.647491781698080970, 185.3224403731376810, 308.0171747953146451 ) ) ;
#20165=PRODUCT ( 'Handle Handwheel Knob', 'Handle Handwheel Knob', '', ( #21359 ) ) ;
#20176=CARTESIAN_POINT ( 'NONE',  ( 12.56180216312617226, 190.5919383268307286, 307.8320289183637897 ) ) ;
#20177=CARTESIAN_POINT ( 'NONE',  ( -8.967245084563666424, 185.1109935582825869, 305.2095739818239508 ) ) ;
#20189=CARTESIAN_POINT ( 'NONE',  ( -22.66159625276162970, 324.6936785073799001, 307.5691494985305781 ) ) ;
#20199=AXIS2_PLACEMENT_3D ( 'NONE', #19909, #981, #4180 ) ;
#20215=CARTESIAN_POINT ( 'NONE',  ( 3.898201936395599532, 166.6627968962365287, 301.5965304707955852 ) ) ;
#20228=TOROIDAL_SURFACE ( 'NONE', #16235, 8.000000000000001776, 6.520833333333323267 ) ;
#20229=ORIENTED_EDGE ( 'NONE', *, *, #13175, .T. ) ;
#20247=CARTESIAN_POINT ( 'NONE',  ( 18.75241981682919956, 183.8790985612903057, 320.1233202157981168 ) ) ;
#20283=CARTESIAN_POINT ( 'NONE',  ( -12.88085435000319912, 181.6037740665256877, 307.3265075889623290 ) ) ;
#20295=VECTOR ( 'NONE', #5140, 999.9999999999998863 ) ;
#20299=DIRECTION ( 'NONE',  ( 0.9934404589540163366, 0.1135548637187057258, -0.01346653032743021922 ) ) ;
#20303=DIRECTION ( 'NONE',  ( 0.3101392564284315978, 0.9506461370142478273, -0.009250070373107145000 ) ) ;
#20309=AXIS2_PLACEMENT_3D ( 'NONE', #6785, #20795, #12082 ) ;
#20314=ORIENTED_EDGE ( 'NONE', *, *, #6929, .T. ) ;
#20322=CARTESIAN_POINT ( 'NONE',  ( 3.898201936395599532, 166.6627968962365287, 301.5965304707955852 ) ) ;
#20326=CARTESIAN_POINT ( 'NONE',  ( -14.11265002968298177, 325.6970952274145361, 313.9537617855303324 ) ) ;
#20341=EDGE_LOOP ( 'NONE', ( #4044, #13405, #18608, #1996, #10990 ) ) ;
#20357=FACE_OUTER_BOUND ( 'NONE', #21869, .T. ) ;
#20369=CARTESIAN_POINT ( 'NONE',  ( -11.09605440033590185, 186.4570468891244559, 320.9292597536728522 ) ) ;
#20389=PRODUCT_DEFINITION ( 'UNKNOWN', '', #19444, #8563 ) ;
#20390=ORIENTED_EDGE ( 'NONE', *, *, #18322, .F. ) ;
#20392=CARTESIAN_POINT ( 'NONE',  ( -8.664060416302492129, 185.3179921677720472, 305.1700144434819322 ) ) ;
#20402=CARTESIAN_POINT ( 'NONE',  ( -15.22406540918863982, 178.2721462461353497, 317.5143574882988560 ) ) ;
#20405=CARTESIAN_POINT ( 'NONE',  ( -13.92525281995234820, 325.7770340667113942, 328.4523304068723064 ) ) ;
#20412=CARTESIAN_POINT ( 'NONE',  ( -26.33924170010756427, 324.2792865754714171, 309.1008800470122537 ) ) ;
#20425=CARTESIAN_POINT ( 'NONE',  ( 13.66010556627975880, 189.9441383114576922, 320.7762228549422616 ) ) ;
#20442=ORIENTED_EDGE ( 'NONE', *, *, #15024, .F. ) ;
#20463=B_SPLINE_CURVE_WITH_KNOTS ( 'NONE', 3,
 ( #14543, #20013, #10959, #18306 ),
 .UNSPECIFIED., .F., .F.,
 ( 4, 4 ),
 ( 0.000000000000000000, 0.0001183016465591462605 ),
 .UNSPECIFIED. ) ;
#20480=TOROIDAL_SURFACE ( 'NONE', #6558, 25.50000000000000355, 3.000000000000000000 ) ;
#20509=ORIENTED_EDGE ( 'NONE', *, *, #138, .T. ) ;
#20512=CARTESIAN_POINT ( 'NONE',  ( -9.812611130992889841, 187.6968966475756986, 321.1611080588128289 ) ) ;
#20523=CARTESIAN_POINT ( 'NONE',  ( -14.02864438394168722, 325.7329298795136197, 320.4531201330285626 ) ) ;
#20524=CARTESIAN_POINT ( 'NONE',  ( -12.33415390922155019, 182.0798801194594603, 322.4718643837915124 ) ) ;
#20527=CARTESIAN_POINT ( 'NONE',  ( -27.31669362735653905, 324.2032591843751561, 317.9607093345767908 ) ) ;
#20537=CARTESIAN_POINT ( 'NONE',  ( 4.195452682864946325, 166.7895964344300808, 324.5942600080963985 ) ) ;
#20566=ORIENTED_EDGE ( 'NONE', *, *, #8299, .T. ) ;
#20586=B_SPLINE_CURVE_WITH_KNOTS ( 'NONE', 3,
 ( #2677, #13134, #14641, #7944, #4263, #4151, #18086 ),
 .UNSPECIFIED., .F., .F.,
 ( 4, 3, 4 ),
 ( -5.913099621787071171E-08, -6.617444900424221399E-24, 3.076089232683742422E-05 ),
 .UNSPECIFIED. ) ;
#20588=DIRECTION ( 'NONE',  ( 0.9934404589540163366, 0.1135548637187052540, -0.01346653032742946982 ) ) ;
#20612=CARTESIAN_POINT ( 'NONE',  ( -15.30033708903644296, 245.0148258455450616, 307.9133183403766907 ) ) ;
#20617=B_SPLINE_CURVE_WITH_KNOTS ( 'NONE', 3,
 ( #6899, #17381, #18741, #19076, #17257, #11979, #3121, #10369 ),
 .UNSPECIFIED., .F., .F.,
 ( 4, 2, 2, 4 ),
 ( 0.000000000000000000, 0.001196880956175902120, 0.002393761912351804241, 0.004787523824703608481 ),
 .UNSPECIFIED. ) ;
#20631=CARTESIAN_POINT ( 'NONE',  ( 12.53841518797468346, 187.5782767441390035, 322.9588541052213486 ) ) ;
#20639=EDGE_CURVE ( 'NONE', #5010, #19042, #2136, .T. ) ;
#20640=FACE_OUTER_BOUND ( 'NONE', #1248, .T. ) ;
#20650=VECTOR ( 'NONE', #1108, 999.9999999999998863 ) ;
#20653=CARTESIAN_POINT ( 'NONE',  ( -23.29666191406895237, 324.6732912418805768, 320.5140407611397677 ) ) ;
#20660=CARTESIAN_POINT ( 'NONE',  ( -5.380589158003702188, 174.4012695080579078, 324.6770650933424918 ) ) ;
#20668=ORIENTED_EDGE ( 'NONE', *, *, #21833, .T. ) ;
#20685=CIRCLE ( 'NONE', #18852, 20.50000000000000711 ) ;
#20748=CARTESIAN_POINT ( 'NONE',  ( 13.10093069687895095, 187.3512383165488302, 322.9178784991170232 ) ) ;
#20752=DIRECTION ( 'NONE',  ( -0.01292394549866727679, -0.005513023399720742325, -0.9999012842304692006 ) ) ;
#20777=ORIENTED_EDGE ( 'NONE', *, *, #12257, .F. ) ;
#20785=CARTESIAN_POINT ( 'NONE',  ( -4.762299381711034840, 326.7918550596768910, 320.2627991765112938 ) ) ;
#20795=DIRECTION ( 'NONE',  ( 0.01292394549866742078, 0.005513023399720777019, 0.9999012842304693116 ) ) ;
#20799=CARTESIAN_POINT ( 'NONE',  ( -13.99926948760909795, 325.7454604562529425, 322.7258004511344325 ) ) ;
#20828=CARTESIAN_POINT ( 'NONE',  ( 13.04685173701508205, 190.3009448115034843, 320.8498781618246198 ) ) ;
#20830=CARTESIAN_POINT ( 'NONE',  ( 12.84822208535021915, 190.4846235402699790, 307.8504815015369900 ) ) ;
#20854=FACE_OUTER_BOUND ( 'NONE', #3980, .T. ) ;
#20859=CARTESIAN_POINT ( 'NONE',  ( -17.13003694822599954, 316.2264685093712160, 320.5456208367596105 ) ) ;
#20860=CARTESIAN_POINT ( 'NONE',  ( -8.523216527044569446, 185.4125284852929099, 305.1540476800932424 ) ) ;
#20865=B_SPLINE_CURVE_WITH_KNOTS ( 'NONE', 3,
 ( #21106, #15973, #3641, #12163, #21214, #17566, #10438, #1594, #8683, #6751, #10658, #5015, #19148, #20989, #101, #12288, #15510, #7096, #1937, #5243, #7210, #10782, #8929, #15622, #17337, #15734, #5470, #3425, #213, #17812, #14126, #17457, #1708, #14724, #22566, #12044, #12507, #3296, #6976, #19268, #14239, #6857, #8804, #8583, #5359, #10322 ),
 .UNSPECIFIED., .F., .F.,
 ( 4, 2, 2, 2, 2, 2, 2, 2, 2, 2, 2, 2, 2, 2, 2, 2, 2, 2, 2, 2, 2, 2, 4 ),
 ( 0.000000000000000000, 0.0007988346004489777592, 0.001597669200897955518, 0.003195338401795909736, 0.003994173002244886736, 0.004793007602693864604, 0.006390676803591825543, 0.007988346004489785615, 0.009586015205387746554, 0.01118368440628570923, 0.01278135360718367017, 0.01358018820763266105, 0.01437902280808165539, 0.01517785740853064627, 0.01597669200897963715, 0.01757436120987761544, 0.01917203041077558678, 0.01997086501122459154, 0.02076969961167359630, 0.02236736881257176540, 0.02396503801346993451, 0.02476387261391905376, 0.02556270721436816953 ),
 .UNSPECIFIED. ) ;
#20873=EDGE_CURVE ( 'NONE', #21242, #15318, #3090, .T. ) ;
#20876=LINE ( 'NONE', #1067, #18501 ) ;
#20901=CARTESIAN_POINT ( 'NONE',  ( 21.69134381229430275, 168.7570390772204405, 316.3235220979586870 ) ) ;
#20910=ORIENTED_EDGE ( 'NONE', *, *, #6838, .T. ) ;
#20920=AXIS2_PLACEMENT_3D ( 'NONE', #10749, #2232, #9006 ) ;
#20927=CARTESIAN_POINT ( 'NONE',  ( -25.55593907343507709, 324.4110961426445101, 319.5660351319885990 ) ) ;
#20936=DIRECTION ( 'NONE',  ( 0.9506032891036972909, -0.3102281881984320644, -0.01057629388542894074 ) ) ;
#20947=SURFACE_SIDE_STYLE ('',( #6825 ) ) ;
#20969=ORIENTED_EDGE ( 'NONE', *, *, #637, .F. ) ;
#20970=CARTESIAN_POINT ( 'NONE',  ( 12.37946041904351446, 187.6360129020394254, 322.9658423925303055 ) ) ;
#20977=DIRECTION ( 'NONE',  ( 0.3102455404053341415, 0.9506564598521393128, 0.000000000000000000 ) ) ;
#20979=CARTESIAN_POINT ( 'NONE',  ( -10.92051603998877773, 183.4567045018018518, 323.0038140145950933 ) ) ;
#20987=FACE_OUTER_BOUND ( 'NONE', #10431, .T. ) ;
#20989=CARTESIAN_POINT ( 'NONE',  ( 17.48759048301047869, 184.6901107042388048, 307.3088310089726747 ) ) ;
#21022=CARTESIAN_POINT ( 'NONE',  ( 0.005291762159211760297, 327.3029031209191544, 311.7951952913599030 ) ) ;
#21046=CARTESIAN_POINT ( 'NONE',  ( -26.63628795331713661, 324.2466416883012812, 309.4292525024184215 ) ) ;
#21057=CARTESIAN_POINT ( 'NONE',  ( 19.88808155476299433, 183.5654341500644193, 313.6124693336564633 ) ) ;
#21072=CARTESIAN_POINT ( 'NONE',  ( 15.29795320234381251, 186.1234154815347779, 305.8048709493763226 ) ) ;
#21085=B_SPLINE_CURVE_WITH_KNOTS ( 'NONE', 3,
 ( #3027, #15571, #6486, #20369, #13398, #4631, #3139, #10156, #10264, #13727 ),
 .UNSPECIFIED., .F., .F.,
 ( 4, 2, 2, 2, 4 ),
 ( 0.000000000000000000, 0.002118048795477085657, 0.003177073193215628269, 0.003706585392084899792, 0.004236097590954171314 ),
 .UNSPECIFIED. ) ;
#21089=EDGE_LOOP ( 'NONE', ( #14692, #14276, #20390, #21943 ) ) ;
#21090=CARTESIAN_POINT ( 'NONE',  ( 12.91603429844997741, 190.3480582277193776, 320.8611997870096388 ) ) ;
#21091=EDGE_LOOP ( 'NONE', ( #2145, #1740, #19399, #11154 ) ) ;
#21097=ORIENTED_EDGE ( 'NONE', *, *, #5007, .F. ) ;
#21098=CARTESIAN_POINT ( 'NONE',  ( -14.84893071567995904, 180.4293321838713666, 312.3514243336252889 ) ) ;
#21101=CARTESIAN_POINT ( 'NONE',  ( -15.38762379257795665, 178.0062715105021312, 316.6788287982297447 ) ) ;
#21106=CARTESIAN_POINT ( 'NONE',  ( 11.85964614693714836, 187.7423844643599296, 304.8777488482054423 ) ) ;
#21135=CARTESIAN_POINT ( 'NONE',  ( 16.02863756297163178, 168.1280733087994577, 320.9370496218247126 ) ) ;
#21155=CARTESIAN_POINT ( 'NONE',  ( -26.93345542666578751, 324.2139270369915494, 309.7437723479166607 ) ) ;
#21169=DIRECTION ( 'NONE',  ( 0.3101392564284315978, 0.9506461370142478273, -0.009250070373106959384 ) ) ;
#21171=ORIENTED_EDGE ( 'NONE', *, *, #17629, .F. ) ;
#21180=CARTESIAN_POINT ( 'NONE',  ( 17.20553148001535604, 184.8947804991583155, 307.0627613442703137 ) ) ;
#21204=CARTESIAN_POINT ( 'NONE',  ( -9.825094046574873730, 187.6899473416463309, 321.1602656712647104 ) ) ;
#21210=CARTESIAN_POINT ( 'NONE',  ( -10.33748581482210938, 187.5699477589057835, 308.1934098357545508 ) ) ;
#21212=CARTESIAN_POINT ( 'NONE',  ( -4.597416034112115746, 326.7591350836430593, 307.4820788455573961 ) ) ;
#21213=CARTESIAN_POINT ( 'NONE',  ( -14.02470704512671773, 182.1275625653396162, 318.7217756528992254 ) ) ;
#21214=CARTESIAN_POINT ( 'NONE',  ( 13.09166901539544803, 187.2406732805667389, 305.0407694685882802 ) ) ;
#21236=CARTESIAN_POINT ( 'NONE',  ( 21.87694519636252366, 168.7662676875228556, 313.3507060617185402 ) ) ;
#21242=VERTEX_POINT ( 'NONE', #8305 ) ;
#21256=CARTESIAN_POINT ( 'NONE',  ( -27.63336591784069896, 324.1648741128184952, 317.4228176935731085 ) ) ;
#21271=CARTESIAN_POINT ( 'NONE',  ( 19.63457776109410702, 183.9216010738356886, 312.5996499687972232 ) ) ;
#21276=ADVANCED_FACE ( 'NONE', ( #10590 ), #12538, .T. ) ;
#21285=CARTESIAN_POINT ( 'NONE',  ( 16.43553195852968685, 185.4773513502461810, 308.6447355220632858 ) ) ;
#21295=CARTESIAN_POINT ( 'NONE',  ( -8.330024601187750122, 185.3742117612894447, 323.2535488253523681 ) ) ;
#21325=CARTESIAN_POINT ( 'NONE',  ( 18.96584720174124783, 168.4155415818909205, 308.9361215159025278 ) ) ;
#21326=CARTESIAN_POINT ( 'NONE',  ( -13.95945144365540536, 180.1360528412382394, 320.5617120762407808 ) ) ;
#21348=DIRECTION ( 'NONE',  ( 0.1351880940536943077, -0.9908129862407182298, 0.003715578404455049076 ) ) ;
#21359=PRODUCT_CONTEXT ( 'NONE', #12939, 'mechanical' ) ;
#21373=CARTESIAN_POINT ( 'NONE',  ( -22.49358496127895535, 324.7653478115763050, 320.5678661935266973 ) ) ;
#21376=ORIENTED_EDGE ( 'NONE', *, *, #16172, .T. ) ;
#21400=CARTESIAN_POINT ( 'NONE',  ( 16.16886689564234203, 187.9666359398803195, 308.7864178224293710 ) ) ;
#21420=ADVANCED_FACE ( 'NONE', ( #15660 ), #19840, .T. ) ;
#21426=ORIENTED_EDGE ( 'NONE', *, *, #3227, .F. ) ;
#21428=CARTESIAN_POINT ( 'NONE',  ( -13.98112707844397562, 325.7531995422979207, 324.1294444254230598 ) ) ;
#21434=CARTESIAN_POINT ( 'NONE',  ( -8.923556136456276988, 185.7170635346084850, 321.2501826865298540 ) ) ;
#21442=CARTESIAN_POINT ( 'NONE',  ( -15.09688200079015985, 178.5583548832944416, 314.9430077195087847 ) ) ;
#21472=ORIENTED_EDGE ( 'NONE', *, *, #3400, .T. ) ;
#21487=EDGE_CURVE ( 'NONE', #15318, #1967, #20617, .T. ) ;
#21505=CARTESIAN_POINT ( 'NONE',  ( 16.47858955813311965, 187.6702387035254560, 308.9588621408448716 ) ) ;
#21512=FACE_OUTER_BOUND ( 'NONE', #6166, .T. ) ;
#21524=ORIENTED_EDGE ( 'NONE', *, *, #21827, .F. ) ;
#21538=CARTESIAN_POINT ( 'NONE',  ( -15.10727221577994150, 179.7316785371915842, 313.5422839745355645 ) ) ;
#21539=ORIENTED_EDGE ( 'NONE', *, *, #7731, .T. ) ;
#21557=CARTESIAN_POINT ( 'NONE',  ( 12.49496009795829643, 188.8219583466606082, 321.3857951847916183 ) ) ;
#21559=DIRECTION ( 'NONE',  ( 0.9506032891036972909, -0.3102281881984320644, -0.01057629388542894074 ) ) ;
#21563=ADVANCED_FACE ( 'NONE', ( #8721 ), #12932, .T. ) ;
#21571=VERTEX_POINT ( 'NONE', #16238 ) ;
#21585=CARTESIAN_POINT ( 'NONE',  ( -22.61872943466546104, 324.6985644157359729, 307.5651070260664142 ) ) ;
#21612=CARTESIAN_POINT ( 'NONE',  ( 19.24716218600273976, 184.5819132463487904, 316.9868485712452184 ) ) ;
#21615=PRODUCT_DEFINITION_SHAPE ( 'NONE', 'NONE',  #20389 ) ;
#21647=CARTESIAN_POINT ( 'NONE',  ( -14.52510427035945995, 181.2105282831826116, 311.5198460221306505 ) ) ;
#21656=ADVANCED_FACE ( 'NONE', ( #19414 ), #16118, .T. ) ;
#21663=CARTESIAN_POINT ( 'NONE',  ( -14.86391513884368187, 178.8380028225893170, 318.6775144440179020 ) ) ;
#21665=CARTESIAN_POINT ( 'NONE',  ( 12.62171595694235471, 189.1959137912106712, 321.1530085673936696 ) ) ;
#21678=CIRCLE ( 'NONE', #16960, 7.000000000000021316 ) ;
#21689=EDGE_CURVE ( 'NONE', #17055, #2643, #22412, .T. ) ;
#21692=PLANE ( 'NONE',  #1911 ) ;
#21720=CARTESIAN_POINT ( 'NONE',  ( 13.03243690953249612, 190.3745391624070180, 307.8621314096817514 ) ) ;
#21731=CARTESIAN_POINT ( 'NONE',  ( 19.94166477935907622, 183.4991379525720276, 314.2419295910784172 ) ) ;
#21763=CARTESIAN_POINT ( 'NONE',  ( -14.18812936803128189, 179.9703185431055203, 311.0925469625015012 ) ) ;
#21770=CARTESIAN_POINT ( 'NONE',  ( 11.89239805793121363, 187.8969028425499914, 305.8235062411625904 ) ) ;
#21781=CARTESIAN_POINT ( 'NONE',  ( -10.62552804867366518, 183.8325962315270203, 305.7046552162815942 ) ) ;
#21782=ORIENTED_EDGE ( 'NONE', *, *, #17667, .T. ) ;
#21789=ADVANCED_FACE ( 'NONE', ( #6089 ), #21692, .T. ) ;
#21790=CARTESIAN_POINT ( 'NONE',  ( -8.773265341766837366, 185.9468773097319172, 306.9487736168949823 ) ) ;
#21796=ADVANCED_FACE ( 'NONE', ( #16457 ), #13116, .T. ) ;
#21815=ADVANCED_FACE ( 'NONE', ( #826, #16789 ), #11377, .T. ) ;
#21827=EDGE_CURVE ( 'NONE', #5334, #13470, #5188, .T. ) ;
#21833=EDGE_CURVE ( 'NONE', #5334, #19478, #8033, .T. ) ;
#21834=EDGE_LOOP ( 'NONE', ( #13399, #3474, #13615, #933 ) ) ;
#21838=CARTESIAN_POINT ( 'NONE',  ( 18.26914968921775539, 184.2849635139225484, 318.6958977197980971 ) ) ;
#21847=CARTESIAN_POINT ( 'NONE',  ( -16.49317536315907162, 164.3238961432036263, 299.8727917740469593 ) ) ;
#21860=CARTESIAN_POINT ( 'NONE',  ( 2.889559250536359425, 175.2456879812082775, 299.5620475989642841 ) ) ;
#21868=ADVANCED_FACE ( 'NONE', ( #18833 ), #20228, .T. ) ;
#21869=EDGE_LOOP ( 'NONE', ( #19285, #21524, #13909, #20442 ) ) ;
#21871=CARTESIAN_POINT ( 'NONE',  ( -9.537647826102183757, 184.6943640793454904, 308.0092459792239765 ) ) ;
#21879=ADVANCED_FACE ( 'NONE', ( #10111 ), #8365, .T. ) ;
#21882=B_SPLINE_CURVE_WITH_KNOTS ( 'NONE', 3,
 ( #7905, #4222, #18254, #14942, #6068, #21885, #799, #13434, #6182, #11474, #21663, #5951, #20402, #4328, #13207, #9854, #15045, #4561, #12990, #18585, #11249, #11354, #6303, #18361, #19956, #18686, #16434, #22001, #16546, #13328, #7796, #2511, #9515, #4660, #14829, #21781, #2631, #13101, #9643, #20177, #4450, #18481 ),
 .UNSPECIFIED., .F., .F.,
 ( 4, 2, 2, 2, 2, 2, 2, 2, 2, 2, 2, 2, 2, 2, 2, 2, 2, 2, 2, 2, 4 ),
 ( 0.005089968351066945750, 0.006687358310421633728, 0.008284748269776320839, 0.009882138229131007950, 0.01068083320880843651, 0.01147952818848586506, 0.01307691814784075687, 0.01387561312751814033, 0.01467430810719552031, 0.01627169806655027681, 0.01707039304622773312, 0.01786908802590518597, 0.01946647798526022002, 0.02106386794461525408, 0.02266125790397028814, 0.02425864786332531872, 0.02585603782268035278, 0.02745342778203538683, 0.02905081774139042089, 0.02984951272106796047, 0.03064820770074549311 ),
 .UNSPECIFIED. ) ;
#21885=CARTESIAN_POINT ( 'NONE',  ( -13.98211408154155855, 180.1057412711771804, 320.5253968426166580 ) ) ;
#21896=CARTESIAN_POINT ( 'NONE',  ( -9.583079365734665345, 187.2593659366937686, 308.0359405774264587 ) ) ;
#21910=DIRECTION ( 'NONE',  ( 0.9934404589540163366, 0.1135548637187057258, -0.01346653032743036146 ) ) ;
#21929=ORIENTED_EDGE ( 'NONE', *, *, #15326, .T. ) ;
#21943=ORIENTED_EDGE ( 'NONE', *, *, #4897, .F. ) ;
#21946=CARTESIAN_POINT ( 'NONE',  ( 20.36766808887146851, 182.1959104846870616, 311.9746127290063100 ) ) ;
#21952=CARTESIAN_POINT ( 'NONE',  ( -10.00417312871659270, 187.8841867195822601, 308.1584149291320500 ) ) ;
#21986=CIRCLE ( 'NONE', #7718, 20.50000000000000000 ) ;
#21987=CARTESIAN_POINT ( 'NONE',  ( -14.62647227136777595, 179.3338414634184801, 312.0078474254344769 ) ) ;
#22000=CARTESIAN_POINT ( 'NONE',  ( 11.62929739413847408, 187.8579631343771439, 307.7555743005772797 ) ) ;
#22001=CARTESIAN_POINT ( 'NONE',  ( -14.22642941140435191, 179.9086452483393828, 309.1547204902269641 ) ) ;
#22011=CARTESIAN_POINT ( 'NONE',  ( -9.995692194476635706, 187.8898849410517471, 308.1575541326492953 ) ) ;
#22032=VERTEX_POINT ( 'NONE', #9036 ) ;
#22054=DIRECTION ( 'NONE',  ( 0.1351880940536942799, -0.9908129862407182298, 0.003715578404455081168 ) ) ;
#22066=CARTESIAN_POINT ( 'NONE',  ( 17.02725847016130345, 185.2342960137961825, 319.7397003021923183 ) ) ;
#22076=ORIENTED_EDGE ( 'NONE', *, *, #21689, .F. ) ;
#22089=CARTESIAN_POINT ( 'NONE',  ( 12.82909088464482217, 190.5347596758964244, 307.8494772114028137 ) ) ;
#22093=CIRCLE ( 'NONE', #16643, 2.272904689641356057 ) ;
#22102=CARTESIAN_POINT ( 'NONE',  ( -10.39997831424552110, 184.0167981025738868, 305.6179304391126834 ) ) ;
#22125=ORIENTED_EDGE ( 'NONE', *, *, #8787, .T. ) ;
#22127=AXIS2_PLACEMENT_3D ( 'NONE', #3462, #13811, #5165 ) ;
#22139=VECTOR ( 'NONE', #19592, 1000.000000000000000 ) ;
#22143=DIRECTION ( 'NONE',  ( 0.9934404589540163366, 0.1135548637187060866, -0.01346653032743036840 ) ) ;
#22147=DIRECTION ( 'NONE',  ( 0.01292394549866742424, 0.005513023399720750999, 0.9999012842304693116 ) ) ;
#22216=CARTESIAN_POINT ( 'NONE',  ( -8.567848615622622788, 185.3757230055408343, 308.0246556707246555 ) ) ;
#22221=CARTESIAN_POINT ( 'NONE',  ( 12.90877429640450380, 187.4316901411805816, 322.9359145523081338 ) ) ;
#22226=CARTESIAN_POINT ( 'NONE',  ( 15.11311956079721774, 186.4324701009672367, 322.6509164249751507 ) ) ;
#22237=CARTESIAN_POINT ( 'NONE',  ( -11.40735840365379339, 183.0524750669035541, 320.8439791889440471 ) ) ;
#22238=CARTESIAN_POINT ( 'NONE',  ( -9.208521424040398529, 186.6689402014612824, 307.7212088717959659 ) ) ;
#22243=AXIS2_PLACEMENT_3D ( 'NONE', #2744, #2845, #20299 ) ;
#22249=CARTESIAN_POINT ( 'NONE',  ( 13.06622344554902249, 190.2899467973469427, 320.8482495152294405 ) ) ;
#22278=DIRECTION ( 'NONE',  ( -0.01292394549866745720, -0.005513023399720816918, -0.9999012842304692006 ) ) ;
#22283=EDGE_CURVE ( 'NONE', #4020, #9497, #4748, .T. ) ;
#22308=CARTESIAN_POINT ( 'NONE',  ( 12.81503532323078964, 190.4972571607467842, 307.8483445055002221 ) ) ;
#22317=ORIENTED_EDGE ( 'NONE', *, *, #8390, .T. ) ;
#22324=ORIENTED_EDGE ( 'NONE', *, *, #13962, .F. ) ;
#22340=DIRECTION ( 'NONE',  ( 0.01292394549866727679, 0.005513023399720742325, 0.9999012842304692006 ) ) ;
#22361=EDGE_CURVE ( 'NONE', #15351, #5229, #2529, .T. ) ;
#22362=ORIENTED_EDGE ( 'NONE', *, *, #10689, .F. ) ;
#22412=CIRCLE ( 'NONE', #8475, 22.49999999999999645 ) ;
#22446=CARTESIAN_POINT ( 'NONE',  ( -5.731715098087014404, 326.6288426432528240, 307.3396573775339107 ) ) ;
#22449=CARTESIAN_POINT ( 'NONE',  ( 12.62120397054262710, 187.5429183231100012, 322.9525087504210887 ) ) ;
#22457=LINE ( 'NONE', #6748, #2589 ) ;
#22492=VECTOR ( 'NONE', #9571, 1000.000000000000114 ) ;
#22511=EDGE_CURVE ( 'NONE', #18283, #3170, #10319, .T. ) ;
#22535=CARTESIAN_POINT ( 'NONE',  ( 11.80168056336799687, 187.7948655116154555, 307.7666879900542085 ) ) ;
#22551=CARTESIAN_POINT ( 'NONE',  ( -12.86548928906161571, 326.2291019854885121, 410.4442357137708086 ) ) ;
#22566=CARTESIAN_POINT ( 'NONE',  ( 19.77615078807425064, 182.9145900011216668, 318.4299545691768003 ) ) ;
#22596=CARTESIAN_POINT ( 'NONE',  ( 21.04327404614685193, 168.6617636117169070, 311.0793389543180751 ) ) ;
#22615=CARTESIAN_POINT ( 'NONE',  ( 16.33911976870347971, 185.7005718863503319, 320.1529740037655642 ) ) ;
#22616=CARTESIAN_POINT ( 'NONE',  ( -26.82015259287494402, 324.2622591174701938, 318.5097988702426619 ) ) ;
#22636=CARTESIAN_POINT ( 'NONE',  ( 12.82301040887749188, 190.4942272971743478, 307.8488580778642358 ) ) ;
#22644=CARTESIAN_POINT ( 'NONE',  ( -10.07221555630028220, 187.8236846762713981, 308.1657108960777691 ) ) ;
#22652=CARTESIAN_POINT ( 'NONE',  ( -8.330024601187750122, 185.3742117612894447, 323.2535488253523681 ) ) ;
#22663=EDGE_LOOP ( 'NONE', ( #5814, #22324, #12767, #6046 ) ) ;
ENDSEC;
END-ISO-10303-21;
